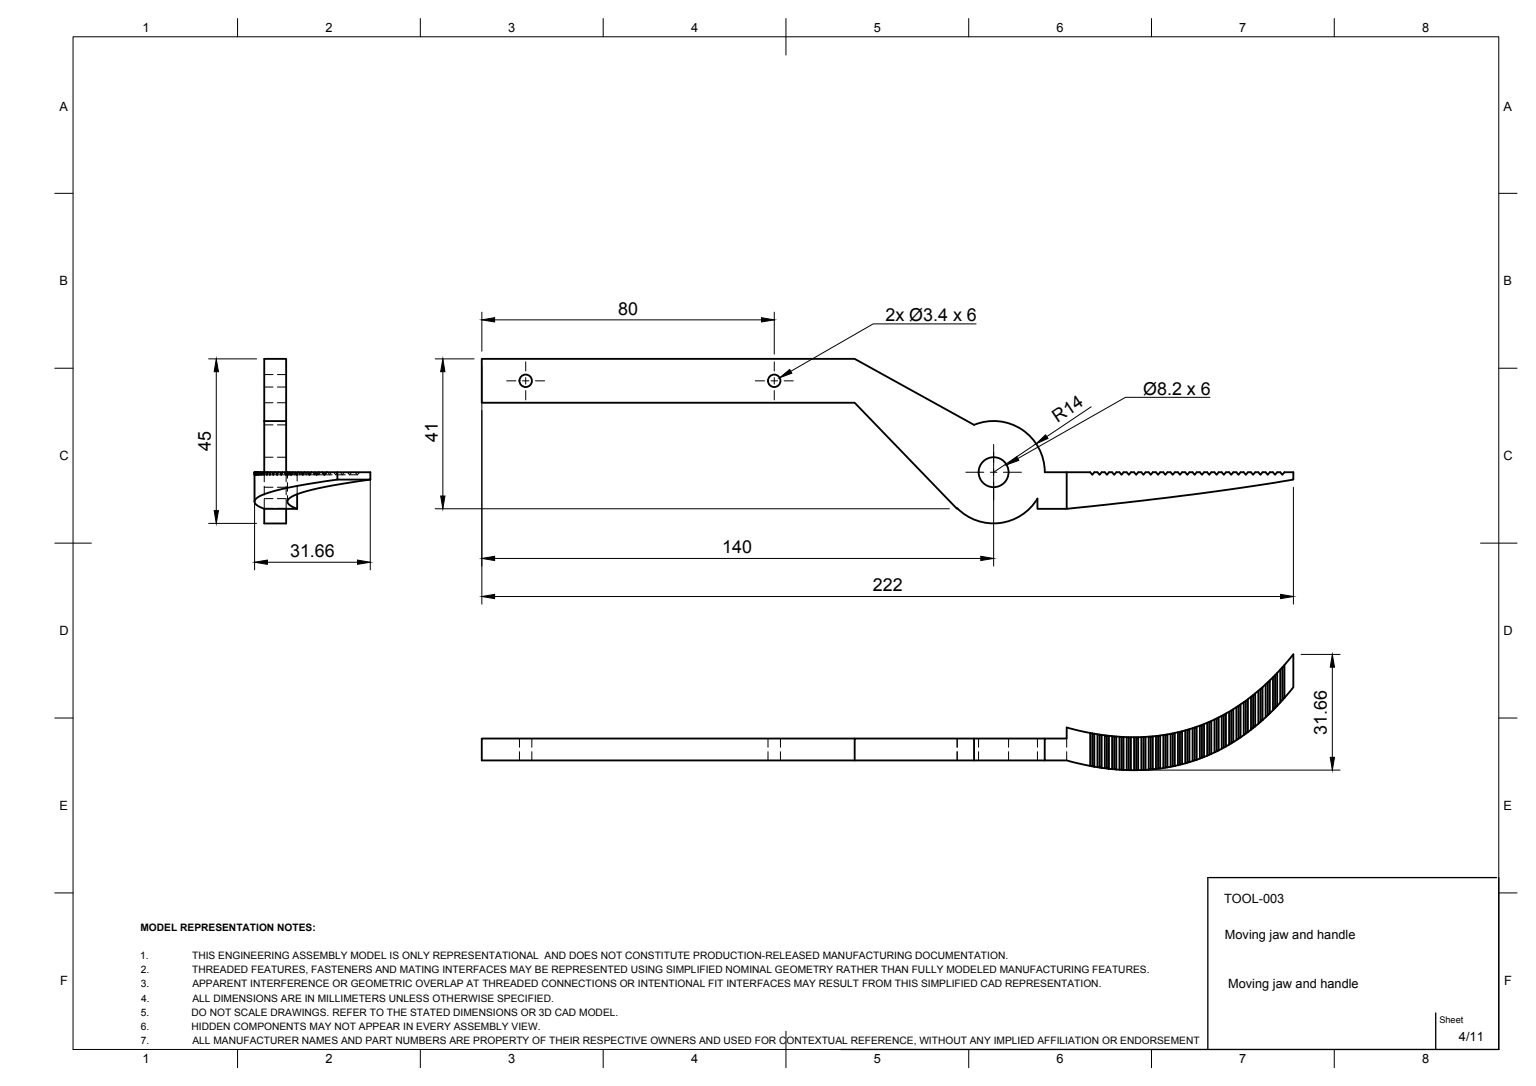
ISO-10303-21;
HEADER;
/* Generated by software containing ST-Developer
 * from STEP Tools, Inc. (www.steptools.com) 
 */

FILE_DESCRIPTION(
/* description */ (''),
/* implementation_level */ '2;1');

FILE_NAME(
/* name */ 'Moving jaw and handle.step',
/* time_stamp */ '2026-11-10T05:20:16-08:00',
/* author */ (''),
/* organization */ (''),
/* preprocessor_version */ 'ST-DEVELOPER v20.2',
/* originating_system */ 'Autodesk Translation Framework v15.17.0.0',
/* authorisation */ '');

FILE_SCHEMA (('AUTOMOTIVE_DESIGN { 1 0 10303 214 3 1 1 }'));
ENDSEC;

DATA;
#10=MECHANICAL_DESIGN_GEOMETRIC_PRESENTATION_REPRESENTATION('',(#113),#24809);
#93=SHAPE_REPRESENTATION_RELATIONSHIP('SRR','None',#24856,#103);
#103=ADVANCED_BREP_SHAPE_REPRESENTATION('',(#123),#24799);
#113=STYLED_ITEM('',(#24919),#123);
#123=MANIFOLD_SOLID_BREP('Body1',#9890);
#138=FACE_BOUND('',#2066,.T.);
#139=FACE_BOUND('',#2067,.T.);
#140=FACE_BOUND('',#2068,.T.);
#141=FACE_BOUND('',#2076,.T.);
#142=FACE_BOUND('',#2077,.T.);
#143=FACE_BOUND('',#2078,.T.);
#202=B_SPLINE_SURFACE_WITH_KNOTS('',3,3,((#14482,#14483,#14484,#14485),
(#14486,#14487,#14488,#14489),(#14490,#14491,#14492,#14493),(#14494,#14495,
#14496,#14497)),.UNSPECIFIED.,.F.,.F.,.F.,(4,4),(4,4),(0.,1.),(0.,1.),
 .UNSPECIFIED.);
#203=B_SPLINE_SURFACE_WITH_KNOTS('',3,3,((#14775,#14776,#14777,#14778),
(#14779,#14780,#14781,#14782),(#14783,#14784,#14785,#14786),(#14787,#14788,
#14789,#14790)),.UNSPECIFIED.,.F.,.F.,.F.,(4,4),(4,4),(0.,1.),(0.,1.),
 .UNSPECIFIED.);
#204=B_SPLINE_SURFACE_WITH_KNOTS('',3,3,((#14799,#14800,#14801,#14802),
(#14803,#14804,#14805,#14806),(#14807,#14808,#14809,#14810),(#14811,#14812,
#14813,#14814)),.UNSPECIFIED.,.F.,.F.,.F.,(4,4),(4,4),(0.,1.),(0.,1.),
 .UNSPECIFIED.);
#451=B_SPLINE_CURVE_WITH_KNOTS('',3,(#13756,#13757,#13758,#13759),
 .UNSPECIFIED.,.F.,.F.,(4,4),(-0.0905761996649145,0.),.UNSPECIFIED.);
#452=B_SPLINE_CURVE_WITH_KNOTS('',3,(#13763,#13764,#13765,#13766),
 .UNSPECIFIED.,.F.,.F.,(4,4),(-0.140808190495876,-0.0502319921300094),
 .UNSPECIFIED.);
#453=B_SPLINE_CURVE_WITH_KNOTS('',3,(#13770,#13771,#13772,#13773),
 .UNSPECIFIED.,.F.,.F.,(4,4),(-0.140839715426601,-0.050218000331002),
 .UNSPECIFIED.);
#454=B_SPLINE_CURVE_WITH_KNOTS('',3,(#13776,#13777,#13778,#13779),
 .UNSPECIFIED.,.F.,.F.,(4,4),(-0.0906217137909262,0.),.UNSPECIFIED.);
#455=B_SPLINE_CURVE_WITH_KNOTS('',3,(#13783,#13784,#13785,#13786),
 .UNSPECIFIED.,.F.,.F.,(4,4),(-0.0903212873282921,0.),.UNSPECIFIED.);
#456=B_SPLINE_CURVE_WITH_KNOTS('',3,(#13790,#13791,#13792,#13793),
 .UNSPECIFIED.,.F.,.F.,(4,4),(-0.140404708440305,-0.0500834223435583),
 .UNSPECIFIED.);
#457=B_SPLINE_CURVE_WITH_KNOTS('',3,(#13797,#13798,#13799,#13800),
 .UNSPECIFIED.,.F.,.F.,(4,4),(-0.14042464555609,-0.0500745698464118),
 .UNSPECIFIED.);
#458=B_SPLINE_CURVE_WITH_KNOTS('',3,(#13803,#13804,#13805,#13806),
 .UNSPECIFIED.,.F.,.F.,(4,4),(-0.0903500744707045,0.),.UNSPECIFIED.);
#459=B_SPLINE_CURVE_WITH_KNOTS('',3,(#13810,#13811,#13812,#13813),
 .UNSPECIFIED.,.F.,.F.,(4,4),(-0.0901993320901174,0.),.UNSPECIFIED.);
#460=B_SPLINE_CURVE_WITH_KNOTS('',3,(#13817,#13818,#13819,#13820),
 .UNSPECIFIED.,.F.,.F.,(4,4),(-0.140206191642939,-0.0500068606873887),
 .UNSPECIFIED.);
#461=B_SPLINE_CURVE_WITH_KNOTS('',3,(#13824,#13825,#13826,#13827),
 .UNSPECIFIED.,.F.,.F.,(4,4),(-0.14021182661721,-0.0500043514612263),
 .UNSPECIFIED.);
#462=B_SPLINE_CURVE_WITH_KNOTS('',3,(#13830,#13831,#13832,#13833),
 .UNSPECIFIED.,.F.,.F.,(4,4),(-0.0902074740142199,0.),.UNSPECIFIED.);
#463=B_SPLINE_CURVE_WITH_KNOTS('',3,(#13837,#13838,#13839,#13840),
 .UNSPECIFIED.,.F.,.F.,(4,4),(-0.0902411601010579,0.),.UNSPECIFIED.);
#464=B_SPLINE_CURVE_WITH_KNOTS('',3,(#13844,#13845,#13846,#13847),
 .UNSPECIFIED.,.F.,.F.,(4,4),(-0.140260192719421,-0.0500190336234041),
 .UNSPECIFIED.);
#465=B_SPLINE_CURVE_WITH_KNOTS('',3,(#13851,#13852,#13853,#13854),
 .UNSPECIFIED.,.F.,.F.,(4,4),(-0.140248231571563,-0.0500243288351115),
 .UNSPECIFIED.);
#466=B_SPLINE_CURVE_WITH_KNOTS('',3,(#13857,#13858,#13859,#13860),
 .UNSPECIFIED.,.F.,.F.,(4,4),(-0.0902239017224492,0.),.UNSPECIFIED.);
#467=B_SPLINE_CURVE_WITH_KNOTS('',3,(#13864,#13865,#13866,#13867),
 .UNSPECIFIED.,.F.,.F.,(4,4),(-0.090484186224837,0.),.UNSPECIFIED.);
#468=B_SPLINE_CURVE_WITH_KNOTS('',3,(#13871,#13872,#13873,#13874),
 .UNSPECIFIED.,.F.,.F.,(4,4),(-0.140624427659317,-0.0501402422817707),
 .UNSPECIFIED.);
#469=B_SPLINE_CURVE_WITH_KNOTS('',3,(#13878,#13879,#13880,#13881),
 .UNSPECIFIED.,.F.,.F.,(4,4),(-0.140590871945081,-0.0501551157110306),
 .UNSPECIFIED.);
#470=B_SPLINE_CURVE_WITH_KNOTS('',3,(#13884,#13885,#13886,#13887),
 .UNSPECIFIED.,.F.,.F.,(4,4),(-0.0904357553781669,0.),.UNSPECIFIED.);
#471=B_SPLINE_CURVE_WITH_KNOTS('',3,(#13891,#13892,#13893,#13894),
 .UNSPECIFIED.,.F.,.F.,(4,4),(-0.090973834374982,0.),.UNSPECIFIED.);
#472=B_SPLINE_CURVE_WITH_KNOTS('',3,(#13898,#13899,#13900,#13901),
 .UNSPECIFIED.,.F.,.F.,(4,4),(-0.141368966615449,-0.0503951329062475),
 .UNSPECIFIED.);
#473=B_SPLINE_CURVE_WITH_KNOTS('',3,(#13905,#13906,#13907,#13908),
 .UNSPECIFIED.,.F.,.F.,(4,4),(-0.141308961367084,-0.0504217384669459),
 .UNSPECIFIED.);
#474=B_SPLINE_CURVE_WITH_KNOTS('',3,(#13911,#13912,#13913,#13914),
 .UNSPECIFIED.,.F.,.F.,(4,4),(-0.0908872222229066,0.),.UNSPECIFIED.);
#475=B_SPLINE_CURVE_WITH_KNOTS('',3,(#13918,#13919,#13920,#13921),
 .UNSPECIFIED.,.F.,.F.,(4,4),(-0.110639644983061,0.),.UNSPECIFIED.);
#476=B_SPLINE_CURVE_WITH_KNOTS('',3,(#13925,#13926,#13927,#13928),
 .UNSPECIFIED.,.F.,.F.,(4,4),(-0.171616644636876,-0.0609769995431898),
 .UNSPECIFIED.);
#477=B_SPLINE_CURVE_WITH_KNOTS('',3,(#13932,#13933,#13934,#13935),
 .UNSPECIFIED.,.F.,.F.,(4,4),(-0.171044536664633,-0.0612308128915547),
 .UNSPECIFIED.);
#478=B_SPLINE_CURVE_WITH_KNOTS('',3,(#13938,#13939,#13940,#13941),
 .UNSPECIFIED.,.F.,.F.,(4,4),(-0.109813723871753,0.),.UNSPECIFIED.);
#479=B_SPLINE_CURVE_WITH_KNOTS('',3,(#13945,#13946,#13947,#13948),
 .UNSPECIFIED.,.F.,.F.,(4,4),(-0.0922945850422147,0.),.UNSPECIFIED.);
#480=B_SPLINE_CURVE_WITH_KNOTS('',3,(#13952,#13953,#13954,#13955),
 .UNSPECIFIED.,.F.,.F.,(4,4),(-0.143389908932554,-0.0510953242730707),
 .UNSPECIFIED.);
#481=B_SPLINE_CURVE_WITH_KNOTS('',3,(#13959,#13960,#13961,#13962),
 .UNSPECIFIED.,.F.,.F.,(4,4),(-0.143278783493244,-0.0511446064988726),
 .UNSPECIFIED.);
#482=B_SPLINE_CURVE_WITH_KNOTS('',3,(#13965,#13966,#13967,#13968),
 .UNSPECIFIED.,.F.,.F.,(4,4),(-0.0921341766004976,0.),.UNSPECIFIED.);
#483=B_SPLINE_CURVE_WITH_KNOTS('',3,(#13972,#13973,#13974,#13975),
 .UNSPECIFIED.,.F.,.F.,(4,4),(-0.0936688606535915,0.),.UNSPECIFIED.);
#484=B_SPLINE_CURVE_WITH_KNOTS('',3,(#13979,#13980,#13981,#13982),
 .UNSPECIFIED.,.F.,.F.,(4,4),(-0.145498716334213,-0.0518298558949936),
 .UNSPECIFIED.);
#485=B_SPLINE_CURVE_WITH_KNOTS('',3,(#13986,#13987,#13988,#13989),
 .UNSPECIFIED.,.F.,.F.,(4,4),(-0.145343920697893,-0.0518985113244783),
 .UNSPECIFIED.);
#486=B_SPLINE_CURVE_WITH_KNOTS('',3,(#13992,#13993,#13994,#13995),
 .UNSPECIFIED.,.F.,.F.,(4,4),(-0.0934454091497814,0.),.UNSPECIFIED.);
#487=B_SPLINE_CURVE_WITH_KNOTS('',3,(#13999,#14000,#14001,#14002),
 .UNSPECIFIED.,.F.,.F.,(4,4),(-0.0955408943961818,0.),.UNSPECIFIED.);
#488=B_SPLINE_CURVE_WITH_KNOTS('',3,(#14006,#14007,#14008,#14009),
 .UNSPECIFIED.,.F.,.F.,(4,4),(-0.148375189783694,-0.0528342954751738),
 .UNSPECIFIED.);
#489=B_SPLINE_CURVE_WITH_KNOTS('',3,(#14013,#14014,#14015,#14016),
 .UNSPECIFIED.,.F.,.F.,(4,4),(-0.148167070467038,-0.0529266079685813),
 .UNSPECIFIED.);
#490=B_SPLINE_CURVE_WITH_KNOTS('',3,(#14019,#14020,#14021,#14022),
 .UNSPECIFIED.,.F.,.F.,(4,4),(-0.0952404624045437,0.),.UNSPECIFIED.);
#491=B_SPLINE_CURVE_WITH_KNOTS('',3,(#14026,#14027,#14028,#14029),
 .UNSPECIFIED.,.F.,.F.,(4,4),(-0.0980208974210048,0.),.UNSPECIFIED.);
#492=B_SPLINE_CURVE_WITH_KNOTS('',3,(#14033,#14034,#14035,#14036),
 .UNSPECIFIED.,.F.,.F.,(4,4),(-0.152189280292737,-0.0541683828893004),
 .UNSPECIFIED.);
#493=B_SPLINE_CURVE_WITH_KNOTS('',3,(#14040,#14041,#14042,#14043),
 .UNSPECIFIED.,.F.,.F.,(4,4),(-0.151916008013229,-0.0542896020155086),
 .UNSPECIFIED.);
#494=B_SPLINE_CURVE_WITH_KNOTS('',3,(#14046,#14047,#14048,#14049),
 .UNSPECIFIED.,.F.,.F.,(4,4),(-0.0976264059776055,0.),.UNSPECIFIED.);
#495=B_SPLINE_CURVE_WITH_KNOTS('',3,(#14053,#14054,#14055,#14056),
 .UNSPECIFIED.,.F.,.F.,(4,4),(-0.101244462273373,0.),.UNSPECIFIED.);
#496=B_SPLINE_CURVE_WITH_KNOTS('',3,(#14060,#14061,#14062,#14063),
 .UNSPECIFIED.,.F.,.F.,(4,4),(-0.157150018704206,-0.0559055564306627),
 .UNSPECIFIED.);
#497=B_SPLINE_CURVE_WITH_KNOTS('',3,(#14067,#14068,#14069,#14070),
 .UNSPECIFIED.,.F.,.F.,(4,4),(-0.156796992217562,-0.056062161879322),
 .UNSPECIFIED.);
#498=B_SPLINE_CURVE_WITH_KNOTS('',3,(#14073,#14074,#14075,#14076),
 .UNSPECIFIED.,.F.,.F.,(4,4),(-0.100734830337421,0.),.UNSPECIFIED.);
#499=B_SPLINE_CURVE_WITH_KNOTS('',3,(#14080,#14081,#14082,#14083),
 .UNSPECIFIED.,.F.,.F.,(4,4),(-0.10537999886802,0.),.UNSPECIFIED.);
#500=B_SPLINE_CURVE_WITH_KNOTS('',3,(#14087,#14088,#14089,#14090),
 .UNSPECIFIED.,.F.,.F.,(4,4),(-0.163516913195776,-0.058136914319678),
 .UNSPECIFIED.);
#501=B_SPLINE_CURVE_WITH_KNOTS('',3,(#14094,#14095,#14096,#14097),
 .UNSPECIFIED.,.F.,.F.,(4,4),(-0.163065906917568,-0.0583369938462544),
 .UNSPECIFIED.);
#502=B_SPLINE_CURVE_WITH_KNOTS('',3,(#14100,#14101,#14102,#14103),
 .UNSPECIFIED.,.F.,.F.,(4,4),(-0.104728913077325,0.),.UNSPECIFIED.);
#503=B_SPLINE_CURVE_WITH_KNOTS('',3,(#14107,#14108,#14109,#14110),
 .UNSPECIFIED.,.F.,.F.,(4,4),(-0.1078539391682,0.),.UNSPECIFIED.);
#504=B_SPLINE_CURVE_WITH_KNOTS('',3,(#14114,#14115,#14116,#14117),
 .UNSPECIFIED.,.F.,.F.,(4,4),(-0.167326517821918,-0.0594725786155369),
 .UNSPECIFIED.);
#505=B_SPLINE_CURVE_WITH_KNOTS('',3,(#14121,#14122,#14123,#14124),
 .UNSPECIFIED.,.F.,.F.,(4,4),(-0.16681822317347,-0.0596980774786193),
 .UNSPECIFIED.);
#506=B_SPLINE_CURVE_WITH_KNOTS('',3,(#14127,#14128,#14129,#14130),
 .UNSPECIFIED.,.F.,.F.,(4,4),(-0.107120145727053,0.),.UNSPECIFIED.);
#507=B_SPLINE_CURVE_WITH_KNOTS('',3,(#14134,#14135,#14136,#14137),
 .UNSPECIFIED.,.F.,.F.,(4,4),(-0.103186160248021,0.),.UNSPECIFIED.);
#508=B_SPLINE_CURVE_WITH_KNOTS('',3,(#14141,#14142,#14143,#14144),
 .UNSPECIFIED.,.F.,.F.,(4,4),(-0.160139097703419,-0.0569529374542383),
 .UNSPECIFIED.);
#509=B_SPLINE_CURVE_WITH_KNOTS('',3,(#14148,#14149,#14150,#14151),
 .UNSPECIFIED.,.F.,.F.,(4,4),(-0.159739629262513,-0.0571301493054397),
 .UNSPECIFIED.);
#510=B_SPLINE_CURVE_WITH_KNOTS('',3,(#14154,#14155,#14156,#14157),
 .UNSPECIFIED.,.F.,.F.,(4,4),(-0.102609479957307,0.),.UNSPECIFIED.);
#511=B_SPLINE_CURVE_WITH_KNOTS('',3,(#14161,#14162,#14163,#14164),
 .UNSPECIFIED.,.F.,.F.,(4,4),(-0.0995300847676173,0.),.UNSPECIFIED.);
#512=B_SPLINE_CURVE_WITH_KNOTS('',3,(#14168,#14169,#14170,#14171),
 .UNSPECIFIED.,.F.,.F.,(4,4),(-0.154511445578318,-0.0549813608126789),
 .UNSPECIFIED.);
#513=B_SPLINE_CURVE_WITH_KNOTS('',3,(#14175,#14176,#14177,#14178),
 .UNSPECIFIED.,.F.,.F.,(4,4),(-0.154200323996305,-0.0551193732220978),
 .UNSPECIFIED.);
#514=B_SPLINE_CURVE_WITH_KNOTS('',3,(#14181,#14182,#14183,#14184),
 .UNSPECIFIED.,.F.,.F.,(4,4),(-0.0990809507692,0.),.UNSPECIFIED.);
#515=B_SPLINE_CURVE_WITH_KNOTS('',3,(#14188,#14189,#14190,#14191),
 .UNSPECIFIED.,.F.,.F.,(4,4),(-0.096697094267499,0.),.UNSPECIFIED.);
#516=B_SPLINE_CURVE_WITH_KNOTS('',3,(#14195,#14196,#14197,#14198),
 .UNSPECIFIED.,.F.,.F.,(4,4),(-0.150152998198254,-0.0534559039759521),
 .UNSPECIFIED.);
#517=B_SPLINE_CURVE_WITH_KNOTS('',3,(#14202,#14203,#14204,#14205),
 .UNSPECIFIED.,.F.,.F.,(4,4),(-0.14991393792459,-0.0535619439725345),
 .UNSPECIFIED.);
#518=B_SPLINE_CURVE_WITH_KNOTS('',3,(#14208,#14209,#14210,#14211),
 .UNSPECIFIED.,.F.,.F.,(4,4),(-0.0963519939024695,0.),.UNSPECIFIED.);
#519=B_SPLINE_CURVE_WITH_KNOTS('',3,(#14215,#14216,#14217,#14218),
 .UNSPECIFIED.,.F.,.F.,(4,4),(-0.0945362942895881,0.),.UNSPECIFIED.);
#520=B_SPLINE_CURVE_WITH_KNOTS('',3,(#14222,#14223,#14224,#14225),
 .UNSPECIFIED.,.F.,.F.,(4,4),(-0.14683118116155,-0.0522948870165077),
 .UNSPECIFIED.);
#521=B_SPLINE_CURVE_WITH_KNOTS('',3,(#14229,#14230,#14231,#14232),
 .UNSPECIFIED.,.F.,.F.,(4,4),(-0.146651054618532,-0.0523747803462794),
 .UNSPECIFIED.);
#522=B_SPLINE_CURVE_WITH_KNOTS('',3,(#14235,#14236,#14237,#14238),
 .UNSPECIFIED.,.F.,.F.,(4,4),(-0.094276274119846,0.),.UNSPECIFIED.);
#523=B_SPLINE_CURVE_WITH_KNOTS('',3,(#14242,#14243,#14244,#14245),
 .UNSPECIFIED.,.F.,.F.,(4,4),(-0.092925555225633,0.),.UNSPECIFIED.);
#524=B_SPLINE_CURVE_WITH_KNOTS('',3,(#14249,#14250,#14251,#14252),
 .UNSPECIFIED.,.F.,.F.,(4,4),(-0.144357688280225,-0.0514321333491983),
 .UNSPECIFIED.);
#525=B_SPLINE_CURVE_WITH_KNOTS('',3,(#14256,#14257,#14258,#14259),
 .UNSPECIFIED.,.F.,.F.,(4,4),(-0.144225816874814,-0.0514906188728281),
 .UNSPECIFIED.);
#526=B_SPLINE_CURVE_WITH_KNOTS('',3,(#14262,#14263,#14264,#14265),
 .UNSPECIFIED.,.F.,.F.,(4,4),(-0.0927351976969034,0.),.UNSPECIFIED.);
#527=B_SPLINE_CURVE_WITH_KNOTS('',3,(#14269,#14270,#14271,#14272),
 .UNSPECIFIED.,.F.,.F.,(4,4),(-0.0917652731638768,0.),.UNSPECIFIED.);
#528=B_SPLINE_CURVE_WITH_KNOTS('',3,(#14276,#14277,#14278,#14279),
 .UNSPECIFIED.,.F.,.F.,(4,4),(-0.142578910435786,-0.0508136377474404),
 .UNSPECIFIED.);
#529=B_SPLINE_CURVE_WITH_KNOTS('',3,(#14283,#14284,#14285,#14286),
 .UNSPECIFIED.,.F.,.F.,(4,4),(-0.142486557842336,-0.0508545922219399),
 .UNSPECIFIED.);
#530=B_SPLINE_CURVE_WITH_KNOTS('',3,(#14289,#14290,#14291,#14292),
 .UNSPECIFIED.,.F.,.F.,(4,4),(-0.0916319651330652,0.),.UNSPECIFIED.);
#531=B_SPLINE_CURVE_WITH_KNOTS('',3,(#14296,#14297,#14298,#14299),
 .UNSPECIFIED.,.F.,.F.,(4,4),(-0.0913279460148378,0.),.UNSPECIFIED.);
#532=B_SPLINE_CURVE_WITH_KNOTS('',3,(#14303,#14304,#14305,#14306),
 .UNSPECIFIED.,.F.,.F.,(4,4),(-0.141909771824219,-0.0505818263802296),
 .UNSPECIFIED.);
#533=B_SPLINE_CURVE_WITH_KNOTS('',3,(#14310,#14311,#14312,#14313),
 .UNSPECIFIED.,.F.,.F.,(4,4),(-0.141834403711857,-0.0506152466388435),
 .UNSPECIFIED.);
#534=B_SPLINE_CURVE_WITH_KNOTS('',3,(#14316,#14317,#14318,#14319),
 .UNSPECIFIED.,.F.,.F.,(4,4),(-0.0912191564904243,0.),.UNSPECIFIED.);
#535=B_SPLINE_CURVE_WITH_KNOTS('',3,(#14323,#14324,#14325,#14326),
 .UNSPECIFIED.,.F.,.F.,(4,4),(-0.0906949857339717,0.),.UNSPECIFIED.);
#536=B_SPLINE_CURVE_WITH_KNOTS('',3,(#14330,#14331,#14332,#14333),
 .UNSPECIFIED.,.F.,.F.,(4,4),(-0.140944227820591,-0.0502492428443703),
 .UNSPECIFIED.);
#537=B_SPLINE_CURVE_WITH_KNOTS('',3,(#14337,#14338,#14339,#14340),
 .UNSPECIFIED.,.F.,.F.,(4,4),(-0.140898114560254,-0.0502696863145455),
 .UNSPECIFIED.);
#538=B_SPLINE_CURVE_WITH_KNOTS('',3,(#14343,#14344,#14345,#14346),
 .UNSPECIFIED.,.F.,.F.,(4,4),(-0.0906284274757685,0.),.UNSPECIFIED.);
#539=B_SPLINE_CURVE_WITH_KNOTS('',3,(#14350,#14351,#14352,#14353),
 .UNSPECIFIED.,.F.,.F.,(4,4),(-0.0903348907359758,0.),.UNSPECIFIED.);
#540=B_SPLINE_CURVE_WITH_KNOTS('',3,(#14357,#14358,#14359,#14360),
 .UNSPECIFIED.,.F.,.F.,(4,4),(-0.140399469840189,-0.0500645800333094),
 .UNSPECIFIED.);
#541=B_SPLINE_CURVE_WITH_KNOTS('',3,(#14364,#14365,#14366,#14367),
 .UNSPECIFIED.,.F.,.F.,(4,4),(-0.140377260822424,-0.0500744206159611),
 .UNSPECIFIED.);
#542=B_SPLINE_CURVE_WITH_KNOTS('',3,(#14370,#14371,#14372,#14373),
 .UNSPECIFIED.,.F.,.F.,(4,4),(-0.0903028392675632,0.),.UNSPECIFIED.);
#543=B_SPLINE_CURVE_WITH_KNOTS('',3,(#14377,#14378,#14379,#14380),
 .UNSPECIFIED.,.F.,.F.,(4,4),(-0.0901976044608984,0.),.UNSPECIFIED.);
#544=B_SPLINE_CURVE_WITH_KNOTS('',3,(#14384,#14385,#14386,#14387),
 .UNSPECIFIED.,.F.,.F.,(4,4),(-0.140198281967887,-0.050000678580588),
 .UNSPECIFIED.);
#545=B_SPLINE_CURVE_WITH_KNOTS('',3,(#14391,#14392,#14393,#14394),
 .UNSPECIFIED.,.F.,.F.,(4,4),(-0.14019557144157,-0.0500018708171553),
 .UNSPECIFIED.);
#546=B_SPLINE_CURVE_WITH_KNOTS('',3,(#14397,#14398,#14399,#14400),
 .UNSPECIFIED.,.F.,.F.,(4,4),(-0.0901936995426637,0.),.UNSPECIFIED.);
#547=B_SPLINE_CURVE_WITH_KNOTS('',3,(#14404,#14405,#14406,#14407),
 .UNSPECIFIED.,.F.,.F.,(4,4),(-0.090241903072294,0.),.UNSPECIFIED.);
#548=B_SPLINE_CURVE_WITH_KNOTS('',3,(#14411,#14412,#14413,#14414),
 .UNSPECIFIED.,.F.,.F.,(4,4),(-0.140277072739373,-0.0500351708536283),
 .UNSPECIFIED.);
#549=B_SPLINE_CURVE_WITH_KNOTS('',3,(#14418,#14419,#14420,#14421),
 .UNSPECIFIED.,.F.,.F.,(4,4),(-0.14029023165943,-0.0500293245949378),
 .UNSPECIFIED.);
#550=B_SPLINE_CURVE_WITH_KNOTS('',3,(#14424,#14425,#14426,#14427),
 .UNSPECIFIED.,.F.,.F.,(4,4),(-0.0902609058696926,0.),.UNSPECIFIED.);
#551=B_SPLINE_CURVE_WITH_KNOTS('',3,(#14431,#14432,#14433,#14434),
 .UNSPECIFIED.,.F.,.F.,(4,4),(-0.0904338265476047,0.),.UNSPECIFIED.);
#552=B_SPLINE_CURVE_WITH_KNOTS('',3,(#14438,#14439,#14440,#14441),
 .UNSPECIFIED.,.F.,.F.,(4,4),(-0.140583455402597,-0.050149630123983),
 .UNSPECIFIED.);
#553=B_SPLINE_CURVE_WITH_KNOTS('',3,(#14445,#14446,#14447,#14448),
 .UNSPECIFIED.,.F.,.F.,(4,4),(-0.140609493729256,-0.0501380716718544),
 .UNSPECIFIED.);
#554=B_SPLINE_CURVE_WITH_KNOTS('',3,(#14451,#14452,#14453,#14454),
 .UNSPECIFIED.,.F.,.F.,(4,4),(-0.0904714207818447,0.),.UNSPECIFIED.);
#555=B_SPLINE_CURVE_WITH_KNOTS('',3,(#14458,#14459,#14460,#14461),
 .UNSPECIFIED.,.F.,.F.,(4,4),(-0.0907453915343808,0.),.UNSPECIFIED.);
#556=B_SPLINE_CURVE_WITH_KNOTS('',3,(#14465,#14466,#14467,#14468),
 .UNSPECIFIED.,.F.,.F.,(4,4),(-0.141074262480741,-0.0503288722684034),
 .UNSPECIFIED.);
#557=B_SPLINE_CURVE_WITH_KNOTS('',3,(#14472,#14473,#14474,#14475),
 .UNSPECIFIED.,.F.,.F.,(4,4),(-0.141110715992304,-0.0503126946273584),
 .UNSPECIFIED.);
#558=B_SPLINE_CURVE_WITH_KNOTS('',3,(#14478,#14479,#14480,#14481),
 .UNSPECIFIED.,.F.,.F.,(4,4),(-0.0907980200379908,0.),.UNSPECIFIED.);
#559=B_SPLINE_CURVE_WITH_KNOTS('',3,(#14498,#14499,#14500,#14501),
 .UNSPECIFIED.,.F.,.F.,(4,4),(0.129763535305857,0.141771498582774),
 .UNSPECIFIED.);
#560=B_SPLINE_CURVE_WITH_KNOTS('',3,(#14502,#14503,#14504,#14505),
 .UNSPECIFIED.,.F.,.F.,(4,4),(0.157691595007123,0.169827160768426),
 .UNSPECIFIED.);
#561=B_SPLINE_CURVE_WITH_KNOTS('',3,(#14506,#14507,#14508,#14509),
 .UNSPECIFIED.,.F.,.F.,(4,4),(0.185918250377541,0.198185574966566),
 .UNSPECIFIED.);
#562=B_SPLINE_CURVE_WITH_KNOTS('',3,(#14510,#14511,#14512,#14513),
 .UNSPECIFIED.,.F.,.F.,(4,4),(0.214453288668711,0.226856759081898),
 .UNSPECIFIED.);
#563=B_SPLINE_CURVE_WITH_KNOTS('',3,(#14514,#14515,#14516,#14517),
 .UNSPECIFIED.,.F.,.F.,(4,4),(0.243307043781977,0.255851295996116),
 .UNSPECIFIED.);
#564=B_SPLINE_CURVE_WITH_KNOTS('',3,(#14518,#14519,#14520,#14521),
 .UNSPECIFIED.,.F.,.F.,(4,4),(0.272490439993122,0.28518037920845),
 .UNSPECIFIED.);
#565=B_SPLINE_CURVE_WITH_KNOTS('',3,(#14522,#14523,#14524,#14525),
 .UNSPECIFIED.,.F.,.F.,(4,4),(0.302015040279167,0.314855863328957),
 .UNSPECIFIED.);
#566=B_SPLINE_CURVE_WITH_KNOTS('',3,(#14526,#14527,#14528,#14529),
 .UNSPECIFIED.,.F.,.F.,(4,4),(0.33189309985356,0.344890320070497),
 .UNSPECIFIED.);
#567=B_SPLINE_CURVE_WITH_KNOTS('',3,(#14530,#14531,#14532,#14533),
 .UNSPECIFIED.,.F.,.F.,(4,4),(0.362137625612687,0.375297100489449),
 .UNSPECIFIED.);
#568=B_SPLINE_CURVE_WITH_KNOTS('',3,(#14534,#14535,#14536,#14537),
 .UNSPECIFIED.,.F.,.F.,(4,4),(0.392762442311623,0.406090404349278),
 .UNSPECIFIED.);
#569=B_SPLINE_CURVE_WITH_KNOTS('',3,(#14538,#14539,#14540,#14541),
 .UNSPECIFIED.,.F.,.F.,(4,4),(0.423782266424232,0.437285357629296),
 .UNSPECIFIED.);
#570=B_SPLINE_CURVE_WITH_KNOTS('',3,(#14542,#14543,#14544,#14545),
 .UNSPECIFIED.,.F.,.F.,(4,4),(0.455212788807218,0.468898099379087),
 .UNSPECIFIED.);
#571=B_SPLINE_CURVE_WITH_KNOTS('',3,(#14546,#14547,#14548,#14549),
 .UNSPECIFIED.,.F.,.F.,(4,4),(0.48707076748574,0.500945879333897),
 .UNSPECIFIED.);
#572=B_SPLINE_CURVE_WITH_KNOTS('',3,(#14550,#14551,#14552,#14553),
 .UNSPECIFIED.,.F.,.F.,(4,4),(0.519374132117822,0.533447167966844),
 .UNSPECIFIED.);
#573=B_SPLINE_CURVE_WITH_KNOTS('',3,(#14554,#14555,#14556,#14557),
 .UNSPECIFIED.,.F.,.F.,(4,4),(0.55214210198613,0.566421780971217),
 .UNSPECIFIED.);
#574=B_SPLINE_CURVE_WITH_KNOTS('',3,(#14558,#14559,#14560,#14561),
 .UNSPECIFIED.,.F.,.F.,(4,4),(0.585395319721713,0.599891020555078),
 .UNSPECIFIED.);
#575=B_SPLINE_CURVE_WITH_KNOTS('',3,(#14562,#14563,#14564,#14565),
 .UNSPECIFIED.,.F.,.F.,(4,4),(0.619156003402013,0.633877836409608),
 .UNSPECIFIED.);
#576=B_SPLINE_CURVE_WITH_KNOTS('',3,(#14566,#14567,#14568,#14569),
 .UNSPECIFIED.,.F.,.F.,(4,4),(0.653448120206462,0.668407009806632),
 .UNSPECIFIED.);
#577=B_SPLINE_CURVE_WITH_KNOTS('',3,(#14570,#14571,#14572,#14573),
 .UNSPECIFIED.,.F.,.F.,(4,4),(0.688297585486082,0.703505365021776),
 .UNSPECIFIED.);
#578=B_SPLINE_CURVE_WITH_KNOTS('',3,(#14574,#14575,#14576,#14577),
 .UNSPECIFIED.,.F.,.F.,(4,4),(0.723732491946339,0.739202013210385),
 .UNSPECIFIED.);
#579=B_SPLINE_CURVE_WITH_KNOTS('',3,(#14578,#14579,#14580,#14581),
 .UNSPECIFIED.,.F.,.F.,(4,4),(0.759783374705264,0.775528635040521),
 .UNSPECIFIED.);
#580=B_SPLINE_CURVE_WITH_KNOTS('',3,(#14582,#14583,#14584,#14585),
 .UNSPECIFIED.,.F.,.F.,(4,4),(0.796483519339086,0.812519809888056),
 .UNSPECIFIED.);
#581=B_SPLINE_CURVE_WITH_KNOTS('',3,(#14586,#14587,#14588,#14589),
 .UNSPECIFIED.,.F.,.F.,(4,4),(0.833869321756548,0.850213401327293),
 .UNSPECIFIED.);
#582=B_SPLINE_CURVE_WITH_KNOTS('',3,(#14590,#14591,#14592,#14593),
 .UNSPECIFIED.,.F.,.F.,(4,4),(0.87198071097596,0.888651011150777),
 .UNSPECIFIED.);
#583=B_SPLINE_CURVE_WITH_KNOTS('',3,(#14594,#14595,#14596,#14597),
 .UNSPECIFIED.,.F.,.F.,(4,4),(0.910861648789003,0.927878517423714),
 .UNSPECIFIED.);
#584=B_SPLINE_CURVE_WITH_KNOTS('',3,(#14599,#14600,#14601,#14602),
 .UNSPECIFIED.,.F.,.F.,(4,4),(0.950560724124997,1.),.UNSPECIFIED.);
#585=B_SPLINE_CURVE_WITH_KNOTS('',3,(#14606,#14607,#14608,#14609,#14610,
#14611),.UNSPECIFIED.,.F.,.F.,(4,2,4),(0.,0.510141450492869,1.),
 .UNSPECIFIED.);
#586=B_SPLINE_CURVE_WITH_KNOTS('',3,(#14614,#14615,#14616,#14617),
 .UNSPECIFIED.,.F.,.F.,(4,4),(0.,0.0865309392501863),.UNSPECIFIED.);
#587=B_SPLINE_CURVE_WITH_KNOTS('',3,(#14618,#14619,#14620,#14621),
 .UNSPECIFIED.,.F.,.F.,(4,4),(0.102124791024766,0.114009094135949),
 .UNSPECIFIED.);
#588=B_SPLINE_CURVE_WITH_KNOTS('',3,(#14624,#14625,#14626,#14627),
 .UNSPECIFIED.,.F.,.F.,(4,4),(0.950560724124998,1.),.UNSPECIFIED.);
#589=B_SPLINE_CURVE_WITH_KNOTS('',3,(#14638,#14639,#14640,#14641),
 .UNSPECIFIED.,.F.,.F.,(4,4),(0.,0.0865309392501863),.UNSPECIFIED.);
#590=B_SPLINE_CURVE_WITH_KNOTS('',3,(#14643,#14644,#14645,#14646),
 .UNSPECIFIED.,.F.,.F.,(4,4),(0.129763535305857,0.141771498582774),
 .UNSPECIFIED.);
#591=B_SPLINE_CURVE_WITH_KNOTS('',3,(#14648,#14649,#14650,#14651),
 .UNSPECIFIED.,.F.,.F.,(4,4),(0.185918250377541,0.198185574966566),
 .UNSPECIFIED.);
#592=B_SPLINE_CURVE_WITH_KNOTS('',3,(#14653,#14654,#14655,#14656),
 .UNSPECIFIED.,.F.,.F.,(4,4),(0.243307043781977,0.255851295996116),
 .UNSPECIFIED.);
#593=B_SPLINE_CURVE_WITH_KNOTS('',3,(#14658,#14659,#14660,#14661),
 .UNSPECIFIED.,.F.,.F.,(4,4),(0.302015040279167,0.314855863328958),
 .UNSPECIFIED.);
#594=B_SPLINE_CURVE_WITH_KNOTS('',3,(#14663,#14664,#14665,#14666),
 .UNSPECIFIED.,.F.,.F.,(4,4),(0.362137625612687,0.375297100489449),
 .UNSPECIFIED.);
#595=B_SPLINE_CURVE_WITH_KNOTS('',3,(#14668,#14669,#14670,#14671),
 .UNSPECIFIED.,.F.,.F.,(4,4),(0.423782266424232,0.437285357629297),
 .UNSPECIFIED.);
#596=B_SPLINE_CURVE_WITH_KNOTS('',3,(#14673,#14674,#14675,#14676),
 .UNSPECIFIED.,.F.,.F.,(4,4),(0.455212788807218,0.468898099379087),
 .UNSPECIFIED.);
#597=B_SPLINE_CURVE_WITH_KNOTS('',3,(#14678,#14679,#14680,#14681),
 .UNSPECIFIED.,.F.,.F.,(4,4),(0.519374132117822,0.533447167966844),
 .UNSPECIFIED.);
#598=B_SPLINE_CURVE_WITH_KNOTS('',3,(#14683,#14684,#14685,#14686),
 .UNSPECIFIED.,.F.,.F.,(4,4),(0.585395319721713,0.599891020555078),
 .UNSPECIFIED.);
#599=B_SPLINE_CURVE_WITH_KNOTS('',3,(#14688,#14689,#14690,#14691),
 .UNSPECIFIED.,.F.,.F.,(4,4),(0.653448120206462,0.668407009806632),
 .UNSPECIFIED.);
#600=B_SPLINE_CURVE_WITH_KNOTS('',3,(#14693,#14694,#14695,#14696),
 .UNSPECIFIED.,.F.,.F.,(4,4),(0.723732491946339,0.739202013210385),
 .UNSPECIFIED.);
#601=B_SPLINE_CURVE_WITH_KNOTS('',3,(#14698,#14699,#14700,#14701),
 .UNSPECIFIED.,.F.,.F.,(4,4),(0.796483519339086,0.812519809888056),
 .UNSPECIFIED.);
#602=B_SPLINE_CURVE_WITH_KNOTS('',3,(#14703,#14704,#14705,#14706),
 .UNSPECIFIED.,.F.,.F.,(4,4),(0.87198071097596,0.888651011150777),
 .UNSPECIFIED.);
#603=B_SPLINE_CURVE_WITH_KNOTS('',3,(#14708,#14709,#14710,#14711),
 .UNSPECIFIED.,.F.,.F.,(4,4),(0.833869321756548,0.850213401327293),
 .UNSPECIFIED.);
#604=B_SPLINE_CURVE_WITH_KNOTS('',3,(#14713,#14714,#14715,#14716),
 .UNSPECIFIED.,.F.,.F.,(4,4),(0.759783374705264,0.775528635040521),
 .UNSPECIFIED.);
#605=B_SPLINE_CURVE_WITH_KNOTS('',3,(#14718,#14719,#14720,#14721),
 .UNSPECIFIED.,.F.,.F.,(4,4),(0.688297585486082,0.703505365021776),
 .UNSPECIFIED.);
#606=B_SPLINE_CURVE_WITH_KNOTS('',3,(#14723,#14724,#14725,#14726),
 .UNSPECIFIED.,.F.,.F.,(4,4),(0.619156003402013,0.633877836409608),
 .UNSPECIFIED.);
#607=B_SPLINE_CURVE_WITH_KNOTS('',3,(#14728,#14729,#14730,#14731),
 .UNSPECIFIED.,.F.,.F.,(4,4),(0.55214210198613,0.566421780971217),
 .UNSPECIFIED.);
#608=B_SPLINE_CURVE_WITH_KNOTS('',3,(#14733,#14734,#14735,#14736),
 .UNSPECIFIED.,.F.,.F.,(4,4),(0.48707076748574,0.500945879333897),
 .UNSPECIFIED.);
#609=B_SPLINE_CURVE_WITH_KNOTS('',3,(#14738,#14739,#14740,#14741),
 .UNSPECIFIED.,.F.,.F.,(4,4),(0.910861648789003,0.927878517423714),
 .UNSPECIFIED.);
#610=B_SPLINE_CURVE_WITH_KNOTS('',3,(#14743,#14744,#14745,#14746),
 .UNSPECIFIED.,.F.,.F.,(4,4),(0.392762442311622,0.406090404349278),
 .UNSPECIFIED.);
#611=B_SPLINE_CURVE_WITH_KNOTS('',3,(#14748,#14749,#14750,#14751),
 .UNSPECIFIED.,.F.,.F.,(4,4),(0.33189309985356,0.344890320070497),
 .UNSPECIFIED.);
#612=B_SPLINE_CURVE_WITH_KNOTS('',3,(#14753,#14754,#14755,#14756),
 .UNSPECIFIED.,.F.,.F.,(4,4),(0.272490439993122,0.28518037920845),
 .UNSPECIFIED.);
#613=B_SPLINE_CURVE_WITH_KNOTS('',3,(#14758,#14759,#14760,#14761),
 .UNSPECIFIED.,.F.,.F.,(4,4),(0.21445328866871,0.226856759081898),
 .UNSPECIFIED.);
#614=B_SPLINE_CURVE_WITH_KNOTS('',3,(#14763,#14764,#14765,#14766),
 .UNSPECIFIED.,.F.,.F.,(4,4),(0.157691595007123,0.169827160768426),
 .UNSPECIFIED.);
#615=B_SPLINE_CURVE_WITH_KNOTS('',3,(#14792,#14793,#14794,#14795,#14796,
#14797),.UNSPECIFIED.,.F.,.F.,(4,2,4),(0.,0.510141450492869,1.),
 .UNSPECIFIED.);
#616=B_SPLINE_CURVE_WITH_KNOTS('',3,(#14815,#14816,#14817,#14818),
 .UNSPECIFIED.,.F.,.F.,(4,4),(0.102124791024766,0.114009094135949),
 .UNSPECIFIED.);
#1093=PLANE('',#10131);
#1094=PLANE('',#10132);
#1095=PLANE('',#10133);
#1096=PLANE('',#10134);
#1097=PLANE('',#10135);
#1098=PLANE('',#10136);
#1099=PLANE('',#10137);
#1100=PLANE('',#10138);
#1101=PLANE('',#10139);
#1102=PLANE('',#10140);
#1103=PLANE('',#10141);
#1104=PLANE('',#10142);
#1105=PLANE('',#10143);
#1106=PLANE('',#10144);
#1107=PLANE('',#10145);
#1108=PLANE('',#10146);
#1109=PLANE('',#10147);
#1110=PLANE('',#10148);
#1111=PLANE('',#10149);
#1112=PLANE('',#10150);
#1113=PLANE('',#10151);
#1114=PLANE('',#10152);
#1115=PLANE('',#10153);
#1116=PLANE('',#10154);
#1117=PLANE('',#10155);
#1118=PLANE('',#10156);
#1119=PLANE('',#10157);
#1120=PLANE('',#10158);
#1121=PLANE('',#10159);
#1122=PLANE('',#10160);
#1123=PLANE('',#10161);
#1124=PLANE('',#10162);
#1125=PLANE('',#10163);
#1126=PLANE('',#10164);
#1127=PLANE('',#10165);
#1128=PLANE('',#10166);
#1129=PLANE('',#10167);
#1130=PLANE('',#10168);
#1131=PLANE('',#10169);
#1132=PLANE('',#10170);
#1133=PLANE('',#10171);
#1134=PLANE('',#10172);
#1135=PLANE('',#10173);
#1136=PLANE('',#10174);
#1137=PLANE('',#10175);
#1138=PLANE('',#10176);
#1139=PLANE('',#10177);
#1140=PLANE('',#10178);
#1141=PLANE('',#10179);
#1142=PLANE('',#10180);
#1143=PLANE('',#10181);
#1144=PLANE('',#10182);
#1145=PLANE('',#10183);
#1146=PLANE('',#10184);
#1147=PLANE('',#10185);
#1148=PLANE('',#10186);
#1149=PLANE('',#10187);
#1150=PLANE('',#10188);
#1151=PLANE('',#10189);
#1152=PLANE('',#10190);
#1153=PLANE('',#10191);
#1154=PLANE('',#10192);
#1155=PLANE('',#10193);
#1156=PLANE('',#10194);
#1157=PLANE('',#10195);
#1158=PLANE('',#10196);
#1159=PLANE('',#10197);
#1160=PLANE('',#10198);
#1161=PLANE('',#10199);
#1162=PLANE('',#10200);
#1163=PLANE('',#10201);
#1164=PLANE('',#10202);
#1165=PLANE('',#10203);
#1166=PLANE('',#10204);
#1167=PLANE('',#10205);
#1168=PLANE('',#10206);
#1169=PLANE('',#10207);
#1170=PLANE('',#10208);
#1171=PLANE('',#10209);
#1172=PLANE('',#10210);
#1173=PLANE('',#10211);
#1174=PLANE('',#10212);
#1175=PLANE('',#10213);
#1176=PLANE('',#10214);
#1177=PLANE('',#10215);
#1178=PLANE('',#10216);
#1179=PLANE('',#10223);
#1180=PLANE('',#10224);
#1181=PLANE('',#10225);
#1182=PLANE('',#10226);
#1183=PLANE('',#10227);
#1184=PLANE('',#10228);
#1185=PLANE('',#10229);
#1186=PLANE('',#10230);
#1412=FACE_OUTER_BOUND('',#1971,.T.);
#1413=FACE_OUTER_BOUND('',#1972,.T.);
#1414=FACE_OUTER_BOUND('',#1973,.T.);
#1415=FACE_OUTER_BOUND('',#1974,.T.);
#1416=FACE_OUTER_BOUND('',#1975,.T.);
#1417=FACE_OUTER_BOUND('',#1976,.T.);
#1418=FACE_OUTER_BOUND('',#1977,.T.);
#1419=FACE_OUTER_BOUND('',#1978,.T.);
#1420=FACE_OUTER_BOUND('',#1979,.T.);
#1421=FACE_OUTER_BOUND('',#1980,.T.);
#1422=FACE_OUTER_BOUND('',#1981,.T.);
#1423=FACE_OUTER_BOUND('',#1982,.T.);
#1424=FACE_OUTER_BOUND('',#1983,.T.);
#1425=FACE_OUTER_BOUND('',#1984,.T.);
#1426=FACE_OUTER_BOUND('',#1985,.T.);
#1427=FACE_OUTER_BOUND('',#1986,.T.);
#1428=FACE_OUTER_BOUND('',#1987,.T.);
#1429=FACE_OUTER_BOUND('',#1988,.T.);
#1430=FACE_OUTER_BOUND('',#1989,.T.);
#1431=FACE_OUTER_BOUND('',#1990,.T.);
#1432=FACE_OUTER_BOUND('',#1991,.T.);
#1433=FACE_OUTER_BOUND('',#1992,.T.);
#1434=FACE_OUTER_BOUND('',#1993,.T.);
#1435=FACE_OUTER_BOUND('',#1994,.T.);
#1436=FACE_OUTER_BOUND('',#1995,.T.);
#1437=FACE_OUTER_BOUND('',#1996,.T.);
#1438=FACE_OUTER_BOUND('',#1997,.T.);
#1439=FACE_OUTER_BOUND('',#1998,.T.);
#1440=FACE_OUTER_BOUND('',#1999,.T.);
#1441=FACE_OUTER_BOUND('',#2000,.T.);
#1442=FACE_OUTER_BOUND('',#2001,.T.);
#1443=FACE_OUTER_BOUND('',#2002,.T.);
#1444=FACE_OUTER_BOUND('',#2003,.T.);
#1445=FACE_OUTER_BOUND('',#2004,.T.);
#1446=FACE_OUTER_BOUND('',#2005,.T.);
#1447=FACE_OUTER_BOUND('',#2006,.T.);
#1448=FACE_OUTER_BOUND('',#2007,.T.);
#1449=FACE_OUTER_BOUND('',#2008,.T.);
#1450=FACE_OUTER_BOUND('',#2009,.T.);
#1451=FACE_OUTER_BOUND('',#2010,.T.);
#1452=FACE_OUTER_BOUND('',#2011,.T.);
#1453=FACE_OUTER_BOUND('',#2012,.T.);
#1454=FACE_OUTER_BOUND('',#2013,.T.);
#1455=FACE_OUTER_BOUND('',#2014,.T.);
#1456=FACE_OUTER_BOUND('',#2015,.T.);
#1457=FACE_OUTER_BOUND('',#2016,.T.);
#1458=FACE_OUTER_BOUND('',#2017,.T.);
#1459=FACE_OUTER_BOUND('',#2018,.T.);
#1460=FACE_OUTER_BOUND('',#2019,.T.);
#1461=FACE_OUTER_BOUND('',#2020,.T.);
#1462=FACE_OUTER_BOUND('',#2021,.T.);
#1463=FACE_OUTER_BOUND('',#2022,.T.);
#1464=FACE_OUTER_BOUND('',#2023,.T.);
#1465=FACE_OUTER_BOUND('',#2024,.T.);
#1466=FACE_OUTER_BOUND('',#2025,.T.);
#1467=FACE_OUTER_BOUND('',#2026,.T.);
#1468=FACE_OUTER_BOUND('',#2027,.T.);
#1469=FACE_OUTER_BOUND('',#2028,.T.);
#1470=FACE_OUTER_BOUND('',#2029,.T.);
#1471=FACE_OUTER_BOUND('',#2030,.T.);
#1472=FACE_OUTER_BOUND('',#2031,.T.);
#1473=FACE_OUTER_BOUND('',#2032,.T.);
#1474=FACE_OUTER_BOUND('',#2033,.T.);
#1475=FACE_OUTER_BOUND('',#2034,.T.);
#1476=FACE_OUTER_BOUND('',#2035,.T.);
#1477=FACE_OUTER_BOUND('',#2036,.T.);
#1478=FACE_OUTER_BOUND('',#2037,.T.);
#1479=FACE_OUTER_BOUND('',#2038,.T.);
#1480=FACE_OUTER_BOUND('',#2039,.T.);
#1481=FACE_OUTER_BOUND('',#2040,.T.);
#1482=FACE_OUTER_BOUND('',#2041,.T.);
#1483=FACE_OUTER_BOUND('',#2042,.T.);
#1484=FACE_OUTER_BOUND('',#2043,.T.);
#1485=FACE_OUTER_BOUND('',#2044,.T.);
#1486=FACE_OUTER_BOUND('',#2045,.T.);
#1487=FACE_OUTER_BOUND('',#2046,.T.);
#1488=FACE_OUTER_BOUND('',#2047,.T.);
#1489=FACE_OUTER_BOUND('',#2048,.T.);
#1490=FACE_OUTER_BOUND('',#2049,.T.);
#1491=FACE_OUTER_BOUND('',#2050,.T.);
#1492=FACE_OUTER_BOUND('',#2051,.T.);
#1493=FACE_OUTER_BOUND('',#2052,.T.);
#1494=FACE_OUTER_BOUND('',#2053,.T.);
#1495=FACE_OUTER_BOUND('',#2054,.T.);
#1496=FACE_OUTER_BOUND('',#2055,.T.);
#1497=FACE_OUTER_BOUND('',#2056,.T.);
#1498=FACE_OUTER_BOUND('',#2057,.T.);
#1499=FACE_OUTER_BOUND('',#2058,.T.);
#1500=FACE_OUTER_BOUND('',#2059,.T.);
#1501=FACE_OUTER_BOUND('',#2060,.T.);
#1502=FACE_OUTER_BOUND('',#2061,.T.);
#1503=FACE_OUTER_BOUND('',#2062,.T.);
#1504=FACE_OUTER_BOUND('',#2063,.T.);
#1505=FACE_OUTER_BOUND('',#2064,.T.);
#1506=FACE_OUTER_BOUND('',#2065,.T.);
#1507=FACE_OUTER_BOUND('',#2069,.T.);
#1508=FACE_OUTER_BOUND('',#2070,.T.);
#1509=FACE_OUTER_BOUND('',#2071,.T.);
#1510=FACE_OUTER_BOUND('',#2072,.T.);
#1511=FACE_OUTER_BOUND('',#2073,.T.);
#1512=FACE_OUTER_BOUND('',#2074,.T.);
#1513=FACE_OUTER_BOUND('',#2075,.T.);
#1971=EDGE_LOOP('',(#6853,#6854,#6855,#6856));
#1972=EDGE_LOOP('',(#6857,#6858,#6859,#6860));
#1973=EDGE_LOOP('',(#6861,#6862,#6863,#6864));
#1974=EDGE_LOOP('',(#6865,#6866,#6867,#6868));
#1975=EDGE_LOOP('',(#6869,#6870,#6871,#6872));
#1976=EDGE_LOOP('',(#6873,#6874,#6875,#6876));
#1977=EDGE_LOOP('',(#6877,#6878,#6879,#6880));
#1978=EDGE_LOOP('',(#6881,#6882,#6883,#6884));
#1979=EDGE_LOOP('',(#6885,#6886,#6887,#6888));
#1980=EDGE_LOOP('',(#6889,#6890,#6891,#6892));
#1981=EDGE_LOOP('',(#6893,#6894,#6895,#6896));
#1982=EDGE_LOOP('',(#6897,#6898,#6899,#6900));
#1983=EDGE_LOOP('',(#6901,#6902,#6903,#6904));
#1984=EDGE_LOOP('',(#6905,#6906,#6907,#6908));
#1985=EDGE_LOOP('',(#6909,#6910,#6911,#6912));
#1986=EDGE_LOOP('',(#6913,#6914,#6915,#6916));
#1987=EDGE_LOOP('',(#6917,#6918,#6919,#6920));
#1988=EDGE_LOOP('',(#6921,#6922,#6923,#6924));
#1989=EDGE_LOOP('',(#6925,#6926,#6927,#6928));
#1990=EDGE_LOOP('',(#6929,#6930,#6931,#6932));
#1991=EDGE_LOOP('',(#6933,#6934,#6935,#6936));
#1992=EDGE_LOOP('',(#6937,#6938,#6939,#6940));
#1993=EDGE_LOOP('',(#6941,#6942,#6943,#6944));
#1994=EDGE_LOOP('',(#6945,#6946,#6947,#6948));
#1995=EDGE_LOOP('',(#6949,#6950,#6951,#6952));
#1996=EDGE_LOOP('',(#6953,#6954,#6955,#6956));
#1997=EDGE_LOOP('',(#6957,#6958,#6959,#6960));
#1998=EDGE_LOOP('',(#6961,#6962,#6963,#6964));
#1999=EDGE_LOOP('',(#6965,#6966,#6967,#6968));
#2000=EDGE_LOOP('',(#6969,#6970,#6971,#6972));
#2001=EDGE_LOOP('',(#6973,#6974,#6975,#6976));
#2002=EDGE_LOOP('',(#6977,#6978,#6979,#6980));
#2003=EDGE_LOOP('',(#6981,#6982,#6983,#6984));
#2004=EDGE_LOOP('',(#6985,#6986,#6987,#6988));
#2005=EDGE_LOOP('',(#6989,#6990,#6991,#6992));
#2006=EDGE_LOOP('',(#6993,#6994,#6995,#6996));
#2007=EDGE_LOOP('',(#6997,#6998,#6999,#7000));
#2008=EDGE_LOOP('',(#7001,#7002,#7003,#7004));
#2009=EDGE_LOOP('',(#7005,#7006,#7007,#7008));
#2010=EDGE_LOOP('',(#7009,#7010,#7011,#7012));
#2011=EDGE_LOOP('',(#7013,#7014,#7015,#7016));
#2012=EDGE_LOOP('',(#7017,#7018,#7019,#7020));
#2013=EDGE_LOOP('',(#7021,#7022,#7023,#7024));
#2014=EDGE_LOOP('',(#7025,#7026,#7027,#7028));
#2015=EDGE_LOOP('',(#7029,#7030,#7031,#7032));
#2016=EDGE_LOOP('',(#7033,#7034,#7035,#7036));
#2017=EDGE_LOOP('',(#7037,#7038,#7039,#7040));
#2018=EDGE_LOOP('',(#7041,#7042,#7043,#7044));
#2019=EDGE_LOOP('',(#7045,#7046,#7047,#7048));
#2020=EDGE_LOOP('',(#7049,#7050,#7051,#7052));
#2021=EDGE_LOOP('',(#7053,#7054,#7055,#7056));
#2022=EDGE_LOOP('',(#7057,#7058,#7059,#7060));
#2023=EDGE_LOOP('',(#7061,#7062,#7063,#7064));
#2024=EDGE_LOOP('',(#7065,#7066,#7067,#7068));
#2025=EDGE_LOOP('',(#7069,#7070,#7071,#7072));
#2026=EDGE_LOOP('',(#7073,#7074,#7075,#7076));
#2027=EDGE_LOOP('',(#7077,#7078,#7079,#7080));
#2028=EDGE_LOOP('',(#7081,#7082,#7083,#7084,#7085,#7086,#7087,#7088,#7089,
#7090,#7091,#7092,#7093,#7094,#7095,#7096,#7097,#7098,#7099,#7100,#7101,
#7102,#7103,#7104,#7105,#7106,#7107,#7108,#7109,#7110,#7111,#7112,#7113,
#7114,#7115,#7116,#7117,#7118,#7119,#7120,#7121,#7122,#7123,#7124,#7125,
#7126,#7127,#7128,#7129,#7130,#7131,#7132,#7133,#7134,#7135,#7136,#7137,
#7138,#7139,#7140,#7141,#7142,#7143,#7144,#7145,#7146,#7147,#7148,#7149,
#7150,#7151,#7152,#7153,#7154,#7155,#7156,#7157,#7158,#7159,#7160,#7161,
#7162,#7163,#7164,#7165));
#2029=EDGE_LOOP('',(#7166,#7167,#7168,#7169));
#2030=EDGE_LOOP('',(#7170,#7171,#7172,#7173,#7174,#7175,#7176));
#2031=EDGE_LOOP('',(#7177,#7178,#7179,#7180));
#2032=EDGE_LOOP('',(#7181,#7182,#7183,#7184));
#2033=EDGE_LOOP('',(#7185,#7186,#7187,#7188));
#2034=EDGE_LOOP('',(#7189,#7190,#7191,#7192));
#2035=EDGE_LOOP('',(#7193,#7194,#7195,#7196));
#2036=EDGE_LOOP('',(#7197,#7198,#7199,#7200));
#2037=EDGE_LOOP('',(#7201,#7202,#7203,#7204));
#2038=EDGE_LOOP('',(#7205,#7206,#7207,#7208));
#2039=EDGE_LOOP('',(#7209,#7210,#7211,#7212));
#2040=EDGE_LOOP('',(#7213,#7214,#7215,#7216));
#2041=EDGE_LOOP('',(#7217,#7218,#7219,#7220));
#2042=EDGE_LOOP('',(#7221,#7222,#7223,#7224));
#2043=EDGE_LOOP('',(#7225,#7226,#7227,#7228));
#2044=EDGE_LOOP('',(#7229,#7230,#7231,#7232));
#2045=EDGE_LOOP('',(#7233,#7234,#7235,#7236));
#2046=EDGE_LOOP('',(#7237,#7238,#7239,#7240));
#2047=EDGE_LOOP('',(#7241,#7242,#7243,#7244));
#2048=EDGE_LOOP('',(#7245,#7246,#7247,#7248));
#2049=EDGE_LOOP('',(#7249,#7250,#7251,#7252));
#2050=EDGE_LOOP('',(#7253,#7254,#7255,#7256));
#2051=EDGE_LOOP('',(#7257,#7258,#7259,#7260));
#2052=EDGE_LOOP('',(#7261,#7262,#7263,#7264));
#2053=EDGE_LOOP('',(#7265,#7266,#7267,#7268));
#2054=EDGE_LOOP('',(#7269,#7270,#7271,#7272));
#2055=EDGE_LOOP('',(#7273,#7274,#7275,#7276));
#2056=EDGE_LOOP('',(#7277,#7278,#7279,#7280));
#2057=EDGE_LOOP('',(#7281,#7282,#7283,#7284));
#2058=EDGE_LOOP('',(#7285,#7286,#7287,#7288,#7289));
#2059=EDGE_LOOP('',(#7290,#7291,#7292,#7293,#7294,#7295,#7296,#7297,#7298,
#7299,#7300,#7301,#7302,#7303,#7304,#7305,#7306,#7307,#7308,#7309,#7310,
#7311,#7312,#7313,#7314,#7315,#7316,#7317,#7318,#7319,#7320,#7321,#7322,
#7323,#7324,#7325,#7326,#7327,#7328,#7329,#7330,#7331,#7332,#7333,#7334,
#7335,#7336,#7337,#7338,#7339,#7340,#7341,#7342,#7343,#7344,#7345,#7346,
#7347,#7348,#7349,#7350,#7351,#7352,#7353,#7354,#7355,#7356,#7357,#7358,
#7359,#7360,#7361,#7362,#7363,#7364,#7365,#7366,#7367,#7368,#7369,#7370,
#7371,#7372,#7373,#7374));
#2060=EDGE_LOOP('',(#7375,#7376,#7377,#7378));
#2061=EDGE_LOOP('',(#7379,#7380,#7381,#7382));
#2062=EDGE_LOOP('',(#7383,#7384,#7385,#7386));
#2063=EDGE_LOOP('',(#7387,#7388,#7389,#7390));
#2064=EDGE_LOOP('',(#7391,#7392,#7393,#7394));
#2065=EDGE_LOOP('',(#7395,#7396,#7397,#7398,#7399,#7400,#7401,#7402,#7403,
#7404,#7405,#7406));
#2066=EDGE_LOOP('',(#7407));
#2067=EDGE_LOOP('',(#7408));
#2068=EDGE_LOOP('',(#7409));
#2069=EDGE_LOOP('',(#7410,#7411,#7412,#7413));
#2070=EDGE_LOOP('',(#7414,#7415,#7416,#7417));
#2071=EDGE_LOOP('',(#7418,#7419,#7420,#7421));
#2072=EDGE_LOOP('',(#7422,#7423,#7424,#7425));
#2073=EDGE_LOOP('',(#7426,#7427,#7428,#7429));
#2074=EDGE_LOOP('',(#7430,#7431,#7432,#7433));
#2075=EDGE_LOOP('',(#7434,#7435,#7436,#7437,#7438,#7439,#7440,#7441,#7442,
#7443,#7444,#7445));
#2076=EDGE_LOOP('',(#7446));
#2077=EDGE_LOOP('',(#7447));
#2078=EDGE_LOOP('',(#7448));
#2605=LINE('',#13739,#3193);
#2606=LINE('',#13745,#3194);
#2607=LINE('',#13751,#3195);
#2608=LINE('',#13761,#3196);
#2609=LINE('',#13767,#3197);
#2610=LINE('',#13775,#3198);
#2611=LINE('',#13788,#3199);
#2612=LINE('',#13794,#3200);
#2613=LINE('',#13802,#3201);
#2614=LINE('',#13815,#3202);
#2615=LINE('',#13821,#3203);
#2616=LINE('',#13829,#3204);
#2617=LINE('',#13842,#3205);
#2618=LINE('',#13848,#3206);
#2619=LINE('',#13856,#3207);
#2620=LINE('',#13869,#3208);
#2621=LINE('',#13875,#3209);
#2622=LINE('',#13883,#3210);
#2623=LINE('',#13896,#3211);
#2624=LINE('',#13902,#3212);
#2625=LINE('',#13910,#3213);
#2626=LINE('',#13923,#3214);
#2627=LINE('',#13929,#3215);
#2628=LINE('',#13937,#3216);
#2629=LINE('',#13950,#3217);
#2630=LINE('',#13956,#3218);
#2631=LINE('',#13964,#3219);
#2632=LINE('',#13977,#3220);
#2633=LINE('',#13983,#3221);
#2634=LINE('',#13991,#3222);
#2635=LINE('',#14004,#3223);
#2636=LINE('',#14010,#3224);
#2637=LINE('',#14018,#3225);
#2638=LINE('',#14031,#3226);
#2639=LINE('',#14037,#3227);
#2640=LINE('',#14045,#3228);
#2641=LINE('',#14058,#3229);
#2642=LINE('',#14064,#3230);
#2643=LINE('',#14072,#3231);
#2644=LINE('',#14085,#3232);
#2645=LINE('',#14091,#3233);
#2646=LINE('',#14099,#3234);
#2647=LINE('',#14112,#3235);
#2648=LINE('',#14118,#3236);
#2649=LINE('',#14126,#3237);
#2650=LINE('',#14139,#3238);
#2651=LINE('',#14145,#3239);
#2652=LINE('',#14153,#3240);
#2653=LINE('',#14166,#3241);
#2654=LINE('',#14172,#3242);
#2655=LINE('',#14180,#3243);
#2656=LINE('',#14193,#3244);
#2657=LINE('',#14199,#3245);
#2658=LINE('',#14207,#3246);
#2659=LINE('',#14220,#3247);
#2660=LINE('',#14226,#3248);
#2661=LINE('',#14234,#3249);
#2662=LINE('',#14247,#3250);
#2663=LINE('',#14253,#3251);
#2664=LINE('',#14261,#3252);
#2665=LINE('',#14274,#3253);
#2666=LINE('',#14280,#3254);
#2667=LINE('',#14288,#3255);
#2668=LINE('',#14301,#3256);
#2669=LINE('',#14307,#3257);
#2670=LINE('',#14315,#3258);
#2671=LINE('',#14328,#3259);
#2672=LINE('',#14334,#3260);
#2673=LINE('',#14342,#3261);
#2674=LINE('',#14355,#3262);
#2675=LINE('',#14361,#3263);
#2676=LINE('',#14369,#3264);
#2677=LINE('',#14382,#3265);
#2678=LINE('',#14388,#3266);
#2679=LINE('',#14396,#3267);
#2680=LINE('',#14409,#3268);
#2681=LINE('',#14415,#3269);
#2682=LINE('',#14423,#3270);
#2683=LINE('',#14436,#3271);
#2684=LINE('',#14442,#3272);
#2685=LINE('',#14450,#3273);
#2686=LINE('',#14463,#3274);
#2687=LINE('',#14469,#3275);
#2688=LINE('',#14477,#3276);
#2689=LINE('',#14604,#3277);
#2690=LINE('',#14613,#3278);
#2691=LINE('',#14628,#3279);
#2692=LINE('',#14631,#3280);
#2693=LINE('',#14633,#3281);
#2694=LINE('',#14635,#3282);
#2695=LINE('',#14637,#3283);
#2696=LINE('',#14769,#3284);
#2697=LINE('',#14770,#3285);
#2698=LINE('',#14773,#3286);
#2699=LINE('',#14774,#3287);
#2700=LINE('',#14798,#3288);
#2701=LINE('',#14819,#3289);
#2702=LINE('',#14823,#3290);
#2703=LINE('',#14825,#3291);
#2704=LINE('',#14826,#3292);
#2705=LINE('',#14830,#3293);
#2706=LINE('',#14831,#3294);
#2707=LINE('',#14832,#3295);
#2708=LINE('',#14837,#3296);
#2709=LINE('',#14843,#3297);
#2710=LINE('',#14847,#3298);
#2711=LINE('',#14849,#3299);
#2712=LINE('',#14851,#3300);
#2713=LINE('',#14853,#3301);
#2714=LINE('',#14855,#3302);
#2715=LINE('',#14856,#3303);
#2716=LINE('',#14859,#3304);
#2717=LINE('',#14860,#3305);
#2718=LINE('',#14863,#3306);
#2719=LINE('',#14864,#3307);
#2720=LINE('',#14867,#3308);
#2721=LINE('',#14868,#3309);
#2722=LINE('',#14871,#3310);
#2723=LINE('',#14872,#3311);
#2724=LINE('',#14875,#3312);
#2725=LINE('',#14876,#3313);
#2726=LINE('',#14878,#3314);
#3193=VECTOR('',#11023,0.17);
#3194=VECTOR('',#11030,0.17);
#3195=VECTOR('',#11037,0.41);
#3196=VECTOR('',#11042,1.);
#3197=VECTOR('',#11043,1.);
#3198=VECTOR('',#11046,1.);
#3199=VECTOR('',#11049,1.);
#3200=VECTOR('',#11050,1.);
#3201=VECTOR('',#11053,1.);
#3202=VECTOR('',#11056,1.);
#3203=VECTOR('',#11057,1.);
#3204=VECTOR('',#11060,1.);
#3205=VECTOR('',#11063,1.);
#3206=VECTOR('',#11064,1.);
#3207=VECTOR('',#11067,1.);
#3208=VECTOR('',#11070,1.);
#3209=VECTOR('',#11071,1.);
#3210=VECTOR('',#11074,1.);
#3211=VECTOR('',#11077,1.);
#3212=VECTOR('',#11078,1.);
#3213=VECTOR('',#11081,1.);
#3214=VECTOR('',#11084,1.);
#3215=VECTOR('',#11085,1.);
#3216=VECTOR('',#11088,1.);
#3217=VECTOR('',#11091,1.);
#3218=VECTOR('',#11092,1.);
#3219=VECTOR('',#11095,1.);
#3220=VECTOR('',#11098,1.);
#3221=VECTOR('',#11099,1.);
#3222=VECTOR('',#11102,1.);
#3223=VECTOR('',#11105,1.);
#3224=VECTOR('',#11106,1.);
#3225=VECTOR('',#11109,1.);
#3226=VECTOR('',#11112,1.);
#3227=VECTOR('',#11113,1.);
#3228=VECTOR('',#11116,1.);
#3229=VECTOR('',#11119,1.);
#3230=VECTOR('',#11120,1.);
#3231=VECTOR('',#11123,1.);
#3232=VECTOR('',#11126,1.);
#3233=VECTOR('',#11127,1.);
#3234=VECTOR('',#11130,1.);
#3235=VECTOR('',#11133,1.);
#3236=VECTOR('',#11134,1.);
#3237=VECTOR('',#11137,1.);
#3238=VECTOR('',#11140,1.);
#3239=VECTOR('',#11141,1.);
#3240=VECTOR('',#11144,1.);
#3241=VECTOR('',#11147,1.);
#3242=VECTOR('',#11148,1.);
#3243=VECTOR('',#11151,1.);
#3244=VECTOR('',#11154,1.);
#3245=VECTOR('',#11155,1.);
#3246=VECTOR('',#11158,1.);
#3247=VECTOR('',#11161,1.);
#3248=VECTOR('',#11162,1.);
#3249=VECTOR('',#11165,1.);
#3250=VECTOR('',#11168,1.);
#3251=VECTOR('',#11169,1.);
#3252=VECTOR('',#11172,1.);
#3253=VECTOR('',#11175,1.);
#3254=VECTOR('',#11176,1.);
#3255=VECTOR('',#11179,1.);
#3256=VECTOR('',#11182,1.);
#3257=VECTOR('',#11183,1.);
#3258=VECTOR('',#11186,1.);
#3259=VECTOR('',#11189,1.);
#3260=VECTOR('',#11190,1.);
#3261=VECTOR('',#11193,1.);
#3262=VECTOR('',#11196,1.);
#3263=VECTOR('',#11197,1.);
#3264=VECTOR('',#11200,1.);
#3265=VECTOR('',#11203,1.);
#3266=VECTOR('',#11204,1.);
#3267=VECTOR('',#11207,1.);
#3268=VECTOR('',#11210,1.);
#3269=VECTOR('',#11211,1.);
#3270=VECTOR('',#11214,1.);
#3271=VECTOR('',#11217,1.);
#3272=VECTOR('',#11218,1.);
#3273=VECTOR('',#11221,1.);
#3274=VECTOR('',#11224,1.);
#3275=VECTOR('',#11225,1.);
#3276=VECTOR('',#11228,1.);
#3277=VECTOR('',#11229,1.);
#3278=VECTOR('',#11230,1.);
#3279=VECTOR('',#11233,1.);
#3280=VECTOR('',#11236,1.);
#3281=VECTOR('',#11237,1.);
#3282=VECTOR('',#11238,1.);
#3283=VECTOR('',#11239,1.);
#3284=VECTOR('',#11292,1.);
#3285=VECTOR('',#11293,1.);
#3286=VECTOR('',#11296,1.);
#3287=VECTOR('',#11297,1.);
#3288=VECTOR('',#11298,1.);
#3289=VECTOR('',#11299,1.);
#3290=VECTOR('',#11304,1.);
#3291=VECTOR('',#11305,1.);
#3292=VECTOR('',#11306,1.);
#3293=VECTOR('',#11309,1.);
#3294=VECTOR('',#11310,1.);
#3295=VECTOR('',#11311,1.);
#3296=VECTOR('',#11316,1.);
#3297=VECTOR('',#11323,1.);
#3298=VECTOR('',#11328,1.);
#3299=VECTOR('',#11329,1.);
#3300=VECTOR('',#11330,1.);
#3301=VECTOR('',#11331,1.);
#3302=VECTOR('',#11332,1.);
#3303=VECTOR('',#11333,1.);
#3304=VECTOR('',#11336,1.);
#3305=VECTOR('',#11337,1.);
#3306=VECTOR('',#11340,1.);
#3307=VECTOR('',#11341,1.);
#3308=VECTOR('',#11344,1.);
#3309=VECTOR('',#11345,1.);
#3310=VECTOR('',#11348,1.);
#3311=VECTOR('',#11349,1.);
#3312=VECTOR('',#11352,1.);
#3313=VECTOR('',#11353,1.);
#3314=VECTOR('',#11356,1.);
#3669=CIRCLE('',#10123,0.17);
#3670=CIRCLE('',#10124,0.17);
#3671=CIRCLE('',#10126,0.17);
#3672=CIRCLE('',#10127,0.17);
#3673=CIRCLE('',#10129,0.41);
#3674=CIRCLE('',#10130,0.41);
#3675=CIRCLE('',#10218,1.4);
#3676=CIRCLE('',#10219,1.4);
#3677=CIRCLE('',#10221,1.4);
#3678=CIRCLE('',#10222,1.4);
#4025=VERTEX_POINT('',#13736);
#4026=VERTEX_POINT('',#13738);
#4027=VERTEX_POINT('',#13742);
#4028=VERTEX_POINT('',#13744);
#4029=VERTEX_POINT('',#13748);
#4030=VERTEX_POINT('',#13750);
#4031=VERTEX_POINT('',#13754);
#4032=VERTEX_POINT('',#13755);
#4033=VERTEX_POINT('',#13760);
#4034=VERTEX_POINT('',#13762);
#4035=VERTEX_POINT('',#13769);
#4036=VERTEX_POINT('',#13774);
#4037=VERTEX_POINT('',#13781);
#4038=VERTEX_POINT('',#13782);
#4039=VERTEX_POINT('',#13787);
#4040=VERTEX_POINT('',#13789);
#4041=VERTEX_POINT('',#13796);
#4042=VERTEX_POINT('',#13801);
#4043=VERTEX_POINT('',#13808);
#4044=VERTEX_POINT('',#13809);
#4045=VERTEX_POINT('',#13814);
#4046=VERTEX_POINT('',#13816);
#4047=VERTEX_POINT('',#13823);
#4048=VERTEX_POINT('',#13828);
#4049=VERTEX_POINT('',#13835);
#4050=VERTEX_POINT('',#13836);
#4051=VERTEX_POINT('',#13841);
#4052=VERTEX_POINT('',#13843);
#4053=VERTEX_POINT('',#13850);
#4054=VERTEX_POINT('',#13855);
#4055=VERTEX_POINT('',#13862);
#4056=VERTEX_POINT('',#13863);
#4057=VERTEX_POINT('',#13868);
#4058=VERTEX_POINT('',#13870);
#4059=VERTEX_POINT('',#13877);
#4060=VERTEX_POINT('',#13882);
#4061=VERTEX_POINT('',#13889);
#4062=VERTEX_POINT('',#13890);
#4063=VERTEX_POINT('',#13895);
#4064=VERTEX_POINT('',#13897);
#4065=VERTEX_POINT('',#13904);
#4066=VERTEX_POINT('',#13909);
#4067=VERTEX_POINT('',#13916);
#4068=VERTEX_POINT('',#13917);
#4069=VERTEX_POINT('',#13922);
#4070=VERTEX_POINT('',#13924);
#4071=VERTEX_POINT('',#13931);
#4072=VERTEX_POINT('',#13936);
#4073=VERTEX_POINT('',#13943);
#4074=VERTEX_POINT('',#13944);
#4075=VERTEX_POINT('',#13949);
#4076=VERTEX_POINT('',#13951);
#4077=VERTEX_POINT('',#13958);
#4078=VERTEX_POINT('',#13963);
#4079=VERTEX_POINT('',#13970);
#4080=VERTEX_POINT('',#13971);
#4081=VERTEX_POINT('',#13976);
#4082=VERTEX_POINT('',#13978);
#4083=VERTEX_POINT('',#13985);
#4084=VERTEX_POINT('',#13990);
#4085=VERTEX_POINT('',#13997);
#4086=VERTEX_POINT('',#13998);
#4087=VERTEX_POINT('',#14003);
#4088=VERTEX_POINT('',#14005);
#4089=VERTEX_POINT('',#14012);
#4090=VERTEX_POINT('',#14017);
#4091=VERTEX_POINT('',#14024);
#4092=VERTEX_POINT('',#14025);
#4093=VERTEX_POINT('',#14030);
#4094=VERTEX_POINT('',#14032);
#4095=VERTEX_POINT('',#14039);
#4096=VERTEX_POINT('',#14044);
#4097=VERTEX_POINT('',#14051);
#4098=VERTEX_POINT('',#14052);
#4099=VERTEX_POINT('',#14057);
#4100=VERTEX_POINT('',#14059);
#4101=VERTEX_POINT('',#14066);
#4102=VERTEX_POINT('',#14071);
#4103=VERTEX_POINT('',#14078);
#4104=VERTEX_POINT('',#14079);
#4105=VERTEX_POINT('',#14084);
#4106=VERTEX_POINT('',#14086);
#4107=VERTEX_POINT('',#14093);
#4108=VERTEX_POINT('',#14098);
#4109=VERTEX_POINT('',#14105);
#4110=VERTEX_POINT('',#14106);
#4111=VERTEX_POINT('',#14111);
#4112=VERTEX_POINT('',#14113);
#4113=VERTEX_POINT('',#14120);
#4114=VERTEX_POINT('',#14125);
#4115=VERTEX_POINT('',#14132);
#4116=VERTEX_POINT('',#14133);
#4117=VERTEX_POINT('',#14138);
#4118=VERTEX_POINT('',#14140);
#4119=VERTEX_POINT('',#14147);
#4120=VERTEX_POINT('',#14152);
#4121=VERTEX_POINT('',#14159);
#4122=VERTEX_POINT('',#14160);
#4123=VERTEX_POINT('',#14165);
#4124=VERTEX_POINT('',#14167);
#4125=VERTEX_POINT('',#14174);
#4126=VERTEX_POINT('',#14179);
#4127=VERTEX_POINT('',#14186);
#4128=VERTEX_POINT('',#14187);
#4129=VERTEX_POINT('',#14192);
#4130=VERTEX_POINT('',#14194);
#4131=VERTEX_POINT('',#14201);
#4132=VERTEX_POINT('',#14206);
#4133=VERTEX_POINT('',#14213);
#4134=VERTEX_POINT('',#14214);
#4135=VERTEX_POINT('',#14219);
#4136=VERTEX_POINT('',#14221);
#4137=VERTEX_POINT('',#14228);
#4138=VERTEX_POINT('',#14233);
#4139=VERTEX_POINT('',#14240);
#4140=VERTEX_POINT('',#14241);
#4141=VERTEX_POINT('',#14246);
#4142=VERTEX_POINT('',#14248);
#4143=VERTEX_POINT('',#14255);
#4144=VERTEX_POINT('',#14260);
#4145=VERTEX_POINT('',#14267);
#4146=VERTEX_POINT('',#14268);
#4147=VERTEX_POINT('',#14273);
#4148=VERTEX_POINT('',#14275);
#4149=VERTEX_POINT('',#14282);
#4150=VERTEX_POINT('',#14287);
#4151=VERTEX_POINT('',#14294);
#4152=VERTEX_POINT('',#14295);
#4153=VERTEX_POINT('',#14300);
#4154=VERTEX_POINT('',#14302);
#4155=VERTEX_POINT('',#14309);
#4156=VERTEX_POINT('',#14314);
#4157=VERTEX_POINT('',#14321);
#4158=VERTEX_POINT('',#14322);
#4159=VERTEX_POINT('',#14327);
#4160=VERTEX_POINT('',#14329);
#4161=VERTEX_POINT('',#14336);
#4162=VERTEX_POINT('',#14341);
#4163=VERTEX_POINT('',#14348);
#4164=VERTEX_POINT('',#14349);
#4165=VERTEX_POINT('',#14354);
#4166=VERTEX_POINT('',#14356);
#4167=VERTEX_POINT('',#14363);
#4168=VERTEX_POINT('',#14368);
#4169=VERTEX_POINT('',#14375);
#4170=VERTEX_POINT('',#14376);
#4171=VERTEX_POINT('',#14381);
#4172=VERTEX_POINT('',#14383);
#4173=VERTEX_POINT('',#14390);
#4174=VERTEX_POINT('',#14395);
#4175=VERTEX_POINT('',#14402);
#4176=VERTEX_POINT('',#14403);
#4177=VERTEX_POINT('',#14408);
#4178=VERTEX_POINT('',#14410);
#4179=VERTEX_POINT('',#14417);
#4180=VERTEX_POINT('',#14422);
#4181=VERTEX_POINT('',#14429);
#4182=VERTEX_POINT('',#14430);
#4183=VERTEX_POINT('',#14435);
#4184=VERTEX_POINT('',#14437);
#4185=VERTEX_POINT('',#14444);
#4186=VERTEX_POINT('',#14449);
#4187=VERTEX_POINT('',#14456);
#4188=VERTEX_POINT('',#14457);
#4189=VERTEX_POINT('',#14462);
#4190=VERTEX_POINT('',#14464);
#4191=VERTEX_POINT('',#14471);
#4192=VERTEX_POINT('',#14476);
#4193=VERTEX_POINT('',#14598);
#4194=VERTEX_POINT('',#14603);
#4195=VERTEX_POINT('',#14605);
#4196=VERTEX_POINT('',#14612);
#4197=VERTEX_POINT('',#14623);
#4198=VERTEX_POINT('',#14630);
#4199=VERTEX_POINT('',#14632);
#4200=VERTEX_POINT('',#14634);
#4201=VERTEX_POINT('',#14636);
#4202=VERTEX_POINT('',#14768);
#4203=VERTEX_POINT('',#14772);
#4204=VERTEX_POINT('',#14791);
#4205=VERTEX_POINT('',#14822);
#4206=VERTEX_POINT('',#14824);
#4207=VERTEX_POINT('',#14828);
#4208=VERTEX_POINT('',#14829);
#4209=VERTEX_POINT('',#14834);
#4210=VERTEX_POINT('',#14836);
#4211=VERTEX_POINT('',#14840);
#4212=VERTEX_POINT('',#14842);
#4213=VERTEX_POINT('',#14846);
#4214=VERTEX_POINT('',#14848);
#4215=VERTEX_POINT('',#14850);
#4216=VERTEX_POINT('',#14852);
#4217=VERTEX_POINT('',#14854);
#4218=VERTEX_POINT('',#14858);
#4219=VERTEX_POINT('',#14862);
#4220=VERTEX_POINT('',#14866);
#4221=VERTEX_POINT('',#14870);
#4222=VERTEX_POINT('',#14874);
#5085=EDGE_CURVE('',#4025,#4025,#3669,.T.);
#5086=EDGE_CURVE('',#4025,#4026,#2605,.T.);
#5087=EDGE_CURVE('',#4026,#4026,#3670,.T.);
#5088=EDGE_CURVE('',#4027,#4027,#3671,.T.);
#5089=EDGE_CURVE('',#4027,#4028,#2606,.T.);
#5090=EDGE_CURVE('',#4028,#4028,#3672,.T.);
#5091=EDGE_CURVE('',#4029,#4029,#3673,.T.);
#5092=EDGE_CURVE('',#4029,#4030,#2607,.T.);
#5093=EDGE_CURVE('',#4030,#4030,#3674,.T.);
#5094=EDGE_CURVE('',#4031,#4032,#451,.T.);
#5095=EDGE_CURVE('',#4033,#4031,#2608,.T.);
#5096=EDGE_CURVE('',#4034,#4033,#452,.T.);
#5097=EDGE_CURVE('',#4032,#4034,#2609,.T.);
#5098=EDGE_CURVE('',#4035,#4031,#453,.T.);
#5099=EDGE_CURVE('',#4036,#4035,#2610,.T.);
#5100=EDGE_CURVE('',#4033,#4036,#454,.T.);
#5101=EDGE_CURVE('',#4037,#4038,#455,.T.);
#5102=EDGE_CURVE('',#4039,#4037,#2611,.T.);
#5103=EDGE_CURVE('',#4040,#4039,#456,.T.);
#5104=EDGE_CURVE('',#4038,#4040,#2612,.T.);
#5105=EDGE_CURVE('',#4041,#4037,#457,.T.);
#5106=EDGE_CURVE('',#4042,#4041,#2613,.T.);
#5107=EDGE_CURVE('',#4039,#4042,#458,.T.);
#5108=EDGE_CURVE('',#4043,#4044,#459,.T.);
#5109=EDGE_CURVE('',#4045,#4043,#2614,.T.);
#5110=EDGE_CURVE('',#4046,#4045,#460,.T.);
#5111=EDGE_CURVE('',#4044,#4046,#2615,.T.);
#5112=EDGE_CURVE('',#4047,#4043,#461,.T.);
#5113=EDGE_CURVE('',#4048,#4047,#2616,.T.);
#5114=EDGE_CURVE('',#4045,#4048,#462,.T.);
#5115=EDGE_CURVE('',#4049,#4050,#463,.T.);
#5116=EDGE_CURVE('',#4051,#4049,#2617,.T.);
#5117=EDGE_CURVE('',#4052,#4051,#464,.T.);
#5118=EDGE_CURVE('',#4050,#4052,#2618,.T.);
#5119=EDGE_CURVE('',#4053,#4049,#465,.T.);
#5120=EDGE_CURVE('',#4054,#4053,#2619,.T.);
#5121=EDGE_CURVE('',#4051,#4054,#466,.T.);
#5122=EDGE_CURVE('',#4055,#4056,#467,.T.);
#5123=EDGE_CURVE('',#4057,#4055,#2620,.T.);
#5124=EDGE_CURVE('',#4058,#4057,#468,.T.);
#5125=EDGE_CURVE('',#4056,#4058,#2621,.T.);
#5126=EDGE_CURVE('',#4059,#4055,#469,.T.);
#5127=EDGE_CURVE('',#4060,#4059,#2622,.T.);
#5128=EDGE_CURVE('',#4057,#4060,#470,.T.);
#5129=EDGE_CURVE('',#4061,#4062,#471,.T.);
#5130=EDGE_CURVE('',#4063,#4061,#2623,.T.);
#5131=EDGE_CURVE('',#4064,#4063,#472,.T.);
#5132=EDGE_CURVE('',#4062,#4064,#2624,.T.);
#5133=EDGE_CURVE('',#4065,#4061,#473,.T.);
#5134=EDGE_CURVE('',#4066,#4065,#2625,.T.);
#5135=EDGE_CURVE('',#4063,#4066,#474,.T.);
#5136=EDGE_CURVE('',#4067,#4068,#475,.T.);
#5137=EDGE_CURVE('',#4069,#4067,#2626,.T.);
#5138=EDGE_CURVE('',#4070,#4069,#476,.T.);
#5139=EDGE_CURVE('',#4068,#4070,#2627,.T.);
#5140=EDGE_CURVE('',#4071,#4067,#477,.T.);
#5141=EDGE_CURVE('',#4072,#4071,#2628,.T.);
#5142=EDGE_CURVE('',#4069,#4072,#478,.T.);
#5143=EDGE_CURVE('',#4073,#4074,#479,.T.);
#5144=EDGE_CURVE('',#4075,#4073,#2629,.T.);
#5145=EDGE_CURVE('',#4076,#4075,#480,.T.);
#5146=EDGE_CURVE('',#4074,#4076,#2630,.T.);
#5147=EDGE_CURVE('',#4077,#4073,#481,.T.);
#5148=EDGE_CURVE('',#4078,#4077,#2631,.T.);
#5149=EDGE_CURVE('',#4075,#4078,#482,.T.);
#5150=EDGE_CURVE('',#4079,#4080,#483,.T.);
#5151=EDGE_CURVE('',#4081,#4079,#2632,.T.);
#5152=EDGE_CURVE('',#4082,#4081,#484,.T.);
#5153=EDGE_CURVE('',#4080,#4082,#2633,.T.);
#5154=EDGE_CURVE('',#4083,#4079,#485,.T.);
#5155=EDGE_CURVE('',#4084,#4083,#2634,.T.);
#5156=EDGE_CURVE('',#4081,#4084,#486,.T.);
#5157=EDGE_CURVE('',#4085,#4086,#487,.T.);
#5158=EDGE_CURVE('',#4087,#4085,#2635,.T.);
#5159=EDGE_CURVE('',#4088,#4087,#488,.T.);
#5160=EDGE_CURVE('',#4086,#4088,#2636,.T.);
#5161=EDGE_CURVE('',#4089,#4085,#489,.T.);
#5162=EDGE_CURVE('',#4090,#4089,#2637,.T.);
#5163=EDGE_CURVE('',#4087,#4090,#490,.T.);
#5164=EDGE_CURVE('',#4091,#4092,#491,.T.);
#5165=EDGE_CURVE('',#4093,#4091,#2638,.T.);
#5166=EDGE_CURVE('',#4094,#4093,#492,.T.);
#5167=EDGE_CURVE('',#4092,#4094,#2639,.T.);
#5168=EDGE_CURVE('',#4095,#4091,#493,.T.);
#5169=EDGE_CURVE('',#4096,#4095,#2640,.T.);
#5170=EDGE_CURVE('',#4093,#4096,#494,.T.);
#5171=EDGE_CURVE('',#4097,#4098,#495,.T.);
#5172=EDGE_CURVE('',#4099,#4097,#2641,.T.);
#5173=EDGE_CURVE('',#4100,#4099,#496,.T.);
#5174=EDGE_CURVE('',#4098,#4100,#2642,.T.);
#5175=EDGE_CURVE('',#4101,#4097,#497,.T.);
#5176=EDGE_CURVE('',#4102,#4101,#2643,.T.);
#5177=EDGE_CURVE('',#4099,#4102,#498,.T.);
#5178=EDGE_CURVE('',#4103,#4104,#499,.T.);
#5179=EDGE_CURVE('',#4105,#4103,#2644,.T.);
#5180=EDGE_CURVE('',#4106,#4105,#500,.T.);
#5181=EDGE_CURVE('',#4104,#4106,#2645,.T.);
#5182=EDGE_CURVE('',#4107,#4103,#501,.T.);
#5183=EDGE_CURVE('',#4108,#4107,#2646,.T.);
#5184=EDGE_CURVE('',#4105,#4108,#502,.T.);
#5185=EDGE_CURVE('',#4109,#4110,#503,.T.);
#5186=EDGE_CURVE('',#4111,#4109,#2647,.T.);
#5187=EDGE_CURVE('',#4112,#4111,#504,.T.);
#5188=EDGE_CURVE('',#4110,#4112,#2648,.T.);
#5189=EDGE_CURVE('',#4113,#4109,#505,.T.);
#5190=EDGE_CURVE('',#4114,#4113,#2649,.T.);
#5191=EDGE_CURVE('',#4111,#4114,#506,.T.);
#5192=EDGE_CURVE('',#4115,#4116,#507,.T.);
#5193=EDGE_CURVE('',#4117,#4115,#2650,.T.);
#5194=EDGE_CURVE('',#4118,#4117,#508,.T.);
#5195=EDGE_CURVE('',#4116,#4118,#2651,.T.);
#5196=EDGE_CURVE('',#4119,#4115,#509,.T.);
#5197=EDGE_CURVE('',#4120,#4119,#2652,.T.);
#5198=EDGE_CURVE('',#4117,#4120,#510,.T.);
#5199=EDGE_CURVE('',#4121,#4122,#511,.T.);
#5200=EDGE_CURVE('',#4123,#4121,#2653,.T.);
#5201=EDGE_CURVE('',#4124,#4123,#512,.T.);
#5202=EDGE_CURVE('',#4122,#4124,#2654,.T.);
#5203=EDGE_CURVE('',#4125,#4121,#513,.T.);
#5204=EDGE_CURVE('',#4126,#4125,#2655,.T.);
#5205=EDGE_CURVE('',#4123,#4126,#514,.T.);
#5206=EDGE_CURVE('',#4127,#4128,#515,.T.);
#5207=EDGE_CURVE('',#4129,#4127,#2656,.T.);
#5208=EDGE_CURVE('',#4130,#4129,#516,.T.);
#5209=EDGE_CURVE('',#4128,#4130,#2657,.T.);
#5210=EDGE_CURVE('',#4131,#4127,#517,.T.);
#5211=EDGE_CURVE('',#4132,#4131,#2658,.T.);
#5212=EDGE_CURVE('',#4129,#4132,#518,.T.);
#5213=EDGE_CURVE('',#4133,#4134,#519,.T.);
#5214=EDGE_CURVE('',#4135,#4133,#2659,.T.);
#5215=EDGE_CURVE('',#4136,#4135,#520,.T.);
#5216=EDGE_CURVE('',#4134,#4136,#2660,.T.);
#5217=EDGE_CURVE('',#4137,#4133,#521,.T.);
#5218=EDGE_CURVE('',#4138,#4137,#2661,.T.);
#5219=EDGE_CURVE('',#4135,#4138,#522,.T.);
#5220=EDGE_CURVE('',#4139,#4140,#523,.T.);
#5221=EDGE_CURVE('',#4141,#4139,#2662,.T.);
#5222=EDGE_CURVE('',#4142,#4141,#524,.T.);
#5223=EDGE_CURVE('',#4140,#4142,#2663,.T.);
#5224=EDGE_CURVE('',#4143,#4139,#525,.T.);
#5225=EDGE_CURVE('',#4144,#4143,#2664,.T.);
#5226=EDGE_CURVE('',#4141,#4144,#526,.T.);
#5227=EDGE_CURVE('',#4145,#4146,#527,.T.);
#5228=EDGE_CURVE('',#4147,#4145,#2665,.T.);
#5229=EDGE_CURVE('',#4148,#4147,#528,.T.);
#5230=EDGE_CURVE('',#4146,#4148,#2666,.T.);
#5231=EDGE_CURVE('',#4149,#4145,#529,.T.);
#5232=EDGE_CURVE('',#4150,#4149,#2667,.T.);
#5233=EDGE_CURVE('',#4147,#4150,#530,.T.);
#5234=EDGE_CURVE('',#4151,#4152,#531,.T.);
#5235=EDGE_CURVE('',#4153,#4151,#2668,.T.);
#5236=EDGE_CURVE('',#4154,#4153,#532,.T.);
#5237=EDGE_CURVE('',#4152,#4154,#2669,.T.);
#5238=EDGE_CURVE('',#4155,#4151,#533,.T.);
#5239=EDGE_CURVE('',#4156,#4155,#2670,.T.);
#5240=EDGE_CURVE('',#4153,#4156,#534,.T.);
#5241=EDGE_CURVE('',#4157,#4158,#535,.T.);
#5242=EDGE_CURVE('',#4159,#4157,#2671,.T.);
#5243=EDGE_CURVE('',#4160,#4159,#536,.T.);
#5244=EDGE_CURVE('',#4158,#4160,#2672,.T.);
#5245=EDGE_CURVE('',#4161,#4157,#537,.T.);
#5246=EDGE_CURVE('',#4162,#4161,#2673,.T.);
#5247=EDGE_CURVE('',#4159,#4162,#538,.T.);
#5248=EDGE_CURVE('',#4163,#4164,#539,.T.);
#5249=EDGE_CURVE('',#4165,#4163,#2674,.T.);
#5250=EDGE_CURVE('',#4166,#4165,#540,.T.);
#5251=EDGE_CURVE('',#4164,#4166,#2675,.T.);
#5252=EDGE_CURVE('',#4167,#4163,#541,.T.);
#5253=EDGE_CURVE('',#4168,#4167,#2676,.T.);
#5254=EDGE_CURVE('',#4165,#4168,#542,.T.);
#5255=EDGE_CURVE('',#4169,#4170,#543,.T.);
#5256=EDGE_CURVE('',#4171,#4169,#2677,.T.);
#5257=EDGE_CURVE('',#4172,#4171,#544,.T.);
#5258=EDGE_CURVE('',#4170,#4172,#2678,.T.);
#5259=EDGE_CURVE('',#4173,#4169,#545,.T.);
#5260=EDGE_CURVE('',#4174,#4173,#2679,.T.);
#5261=EDGE_CURVE('',#4171,#4174,#546,.T.);
#5262=EDGE_CURVE('',#4175,#4176,#547,.T.);
#5263=EDGE_CURVE('',#4177,#4175,#2680,.T.);
#5264=EDGE_CURVE('',#4178,#4177,#548,.T.);
#5265=EDGE_CURVE('',#4176,#4178,#2681,.T.);
#5266=EDGE_CURVE('',#4179,#4175,#549,.T.);
#5267=EDGE_CURVE('',#4180,#4179,#2682,.T.);
#5268=EDGE_CURVE('',#4177,#4180,#550,.T.);
#5269=EDGE_CURVE('',#4181,#4182,#551,.T.);
#5270=EDGE_CURVE('',#4183,#4181,#2683,.T.);
#5271=EDGE_CURVE('',#4184,#4183,#552,.T.);
#5272=EDGE_CURVE('',#4182,#4184,#2684,.T.);
#5273=EDGE_CURVE('',#4185,#4181,#553,.T.);
#5274=EDGE_CURVE('',#4186,#4185,#2685,.T.);
#5275=EDGE_CURVE('',#4183,#4186,#554,.T.);
#5276=EDGE_CURVE('',#4187,#4188,#555,.T.);
#5277=EDGE_CURVE('',#4189,#4187,#2686,.T.);
#5278=EDGE_CURVE('',#4190,#4189,#556,.T.);
#5279=EDGE_CURVE('',#4188,#4190,#2687,.T.);
#5280=EDGE_CURVE('',#4191,#4187,#557,.T.);
#5281=EDGE_CURVE('',#4192,#4191,#2688,.T.);
#5282=EDGE_CURVE('',#4189,#4192,#558,.T.);
#5283=EDGE_CURVE('',#4032,#4185,#559,.T.);
#5284=EDGE_CURVE('',#4182,#4041,#560,.T.);
#5285=EDGE_CURVE('',#4038,#4179,#561,.T.);
#5286=EDGE_CURVE('',#4176,#4047,#562,.T.);
#5287=EDGE_CURVE('',#4044,#4173,#563,.T.);
#5288=EDGE_CURVE('',#4170,#4053,#564,.T.);
#5289=EDGE_CURVE('',#4050,#4167,#565,.T.);
#5290=EDGE_CURVE('',#4164,#4059,#566,.T.);
#5291=EDGE_CURVE('',#4056,#4161,#567,.T.);
#5292=EDGE_CURVE('',#4158,#4065,#568,.T.);
#5293=EDGE_CURVE('',#4062,#4155,#569,.T.);
#5294=EDGE_CURVE('',#4152,#4149,#570,.T.);
#5295=EDGE_CURVE('',#4146,#4077,#571,.T.);
#5296=EDGE_CURVE('',#4074,#4143,#572,.T.);
#5297=EDGE_CURVE('',#4140,#4083,#573,.T.);
#5298=EDGE_CURVE('',#4080,#4137,#574,.T.);
#5299=EDGE_CURVE('',#4134,#4089,#575,.T.);
#5300=EDGE_CURVE('',#4086,#4131,#576,.T.);
#5301=EDGE_CURVE('',#4128,#4095,#577,.T.);
#5302=EDGE_CURVE('',#4092,#4125,#578,.T.);
#5303=EDGE_CURVE('',#4122,#4101,#579,.T.);
#5304=EDGE_CURVE('',#4098,#4119,#580,.T.);
#5305=EDGE_CURVE('',#4116,#4107,#581,.T.);
#5306=EDGE_CURVE('',#4104,#4113,#582,.T.);
#5307=EDGE_CURVE('',#4110,#4071,#583,.T.);
#5308=EDGE_CURVE('',#4068,#4193,#584,.T.);
#5309=EDGE_CURVE('',#4193,#4194,#2689,.T.);
#5310=EDGE_CURVE('',#4195,#4194,#585,.T.);
#5311=EDGE_CURVE('',#4196,#4195,#2690,.T.);
#5312=EDGE_CURVE('',#4196,#4191,#586,.T.);
#5313=EDGE_CURVE('',#4188,#4035,#587,.T.);
#5314=EDGE_CURVE('',#4070,#4197,#588,.T.);
#5315=EDGE_CURVE('',#4197,#4193,#2691,.T.);
#5316=EDGE_CURVE('',#4198,#4196,#2692,.T.);
#5317=EDGE_CURVE('',#4199,#4198,#2693,.T.);
#5318=EDGE_CURVE('',#4200,#4199,#2694,.T.);
#5319=EDGE_CURVE('',#4201,#4200,#2695,.T.);
#5320=EDGE_CURVE('',#4201,#4192,#589,.T.);
#5321=EDGE_CURVE('',#4034,#4186,#590,.T.);
#5322=EDGE_CURVE('',#4040,#4180,#591,.T.);
#5323=EDGE_CURVE('',#4046,#4174,#592,.T.);
#5324=EDGE_CURVE('',#4052,#4168,#593,.T.);
#5325=EDGE_CURVE('',#4058,#4162,#594,.T.);
#5326=EDGE_CURVE('',#4064,#4156,#595,.T.);
#5327=EDGE_CURVE('',#4154,#4150,#596,.T.);
#5328=EDGE_CURVE('',#4076,#4144,#597,.T.);
#5329=EDGE_CURVE('',#4082,#4138,#598,.T.);
#5330=EDGE_CURVE('',#4088,#4132,#599,.T.);
#5331=EDGE_CURVE('',#4094,#4126,#600,.T.);
#5332=EDGE_CURVE('',#4100,#4120,#601,.T.);
#5333=EDGE_CURVE('',#4106,#4114,#602,.T.);
#5334=EDGE_CURVE('',#4118,#4108,#603,.T.);
#5335=EDGE_CURVE('',#4124,#4102,#604,.T.);
#5336=EDGE_CURVE('',#4130,#4096,#605,.T.);
#5337=EDGE_CURVE('',#4136,#4090,#606,.T.);
#5338=EDGE_CURVE('',#4142,#4084,#607,.T.);
#5339=EDGE_CURVE('',#4148,#4078,#608,.T.);
#5340=EDGE_CURVE('',#4112,#4072,#609,.T.);
#5341=EDGE_CURVE('',#4160,#4066,#610,.T.);
#5342=EDGE_CURVE('',#4166,#4060,#611,.T.);
#5343=EDGE_CURVE('',#4172,#4054,#612,.T.);
#5344=EDGE_CURVE('',#4178,#4048,#613,.T.);
#5345=EDGE_CURVE('',#4184,#4042,#614,.T.);
#5346=EDGE_CURVE('',#4202,#4197,#2696,.T.);
#5347=EDGE_CURVE('',#4194,#4202,#2697,.T.);
#5348=EDGE_CURVE('',#4198,#4203,#2698,.T.);
#5349=EDGE_CURVE('',#4195,#4203,#2699,.T.);
#5350=EDGE_CURVE('',#4204,#4202,#615,.T.);
#5351=EDGE_CURVE('',#4203,#4204,#2700,.T.);
#5352=EDGE_CURVE('',#4190,#4036,#616,.T.);
#5353=EDGE_CURVE('',#4204,#4201,#2701,.T.);
#5354=EDGE_CURVE('',#4203,#4205,#2702,.T.);
#5355=EDGE_CURVE('',#4206,#4204,#2703,.T.);
#5356=EDGE_CURVE('',#4205,#4206,#2704,.T.);
#5357=EDGE_CURVE('',#4207,#4208,#2705,.T.);
#5358=EDGE_CURVE('',#4205,#4207,#2706,.T.);
#5359=EDGE_CURVE('',#4208,#4206,#2707,.T.);
#5360=EDGE_CURVE('',#4199,#4209,#3675,.T.);
#5361=EDGE_CURVE('',#4209,#4210,#2708,.T.);
#5362=EDGE_CURVE('',#4200,#4210,#3676,.T.);
#5363=EDGE_CURVE('',#4211,#4208,#3677,.T.);
#5364=EDGE_CURVE('',#4211,#4212,#2709,.T.);
#5365=EDGE_CURVE('',#4212,#4207,#3678,.T.);
#5366=EDGE_CURVE('',#4210,#4213,#2710,.T.);
#5367=EDGE_CURVE('',#4213,#4214,#2711,.T.);
#5368=EDGE_CURVE('',#4214,#4215,#2712,.T.);
#5369=EDGE_CURVE('',#4215,#4216,#2713,.T.);
#5370=EDGE_CURVE('',#4216,#4217,#2714,.T.);
#5371=EDGE_CURVE('',#4217,#4211,#2715,.T.);
#5372=EDGE_CURVE('',#4209,#4218,#2716,.T.);
#5373=EDGE_CURVE('',#4218,#4213,#2717,.T.);
#5374=EDGE_CURVE('',#4219,#4217,#2718,.T.);
#5375=EDGE_CURVE('',#4219,#4212,#2719,.T.);
#5376=EDGE_CURVE('',#4220,#4219,#2720,.T.);
#5377=EDGE_CURVE('',#4220,#4216,#2721,.T.);
#5378=EDGE_CURVE('',#4221,#4220,#2722,.T.);
#5379=EDGE_CURVE('',#4221,#4215,#2723,.T.);
#5380=EDGE_CURVE('',#4222,#4221,#2724,.T.);
#5381=EDGE_CURVE('',#4222,#4214,#2725,.T.);
#5382=EDGE_CURVE('',#4218,#4222,#2726,.T.);
#6853=ORIENTED_EDGE('',*,*,#5085,.F.);
#6854=ORIENTED_EDGE('',*,*,#5086,.T.);
#6855=ORIENTED_EDGE('',*,*,#5087,.F.);
#6856=ORIENTED_EDGE('',*,*,#5086,.F.);
#6857=ORIENTED_EDGE('',*,*,#5088,.F.);
#6858=ORIENTED_EDGE('',*,*,#5089,.T.);
#6859=ORIENTED_EDGE('',*,*,#5090,.F.);
#6860=ORIENTED_EDGE('',*,*,#5089,.F.);
#6861=ORIENTED_EDGE('',*,*,#5091,.F.);
#6862=ORIENTED_EDGE('',*,*,#5092,.T.);
#6863=ORIENTED_EDGE('',*,*,#5093,.F.);
#6864=ORIENTED_EDGE('',*,*,#5092,.F.);
#6865=ORIENTED_EDGE('',*,*,#5094,.F.);
#6866=ORIENTED_EDGE('',*,*,#5095,.F.);
#6867=ORIENTED_EDGE('',*,*,#5096,.F.);
#6868=ORIENTED_EDGE('',*,*,#5097,.F.);
#6869=ORIENTED_EDGE('',*,*,#5098,.F.);
#6870=ORIENTED_EDGE('',*,*,#5099,.F.);
#6871=ORIENTED_EDGE('',*,*,#5100,.F.);
#6872=ORIENTED_EDGE('',*,*,#5095,.T.);
#6873=ORIENTED_EDGE('',*,*,#5101,.F.);
#6874=ORIENTED_EDGE('',*,*,#5102,.F.);
#6875=ORIENTED_EDGE('',*,*,#5103,.F.);
#6876=ORIENTED_EDGE('',*,*,#5104,.F.);
#6877=ORIENTED_EDGE('',*,*,#5105,.F.);
#6878=ORIENTED_EDGE('',*,*,#5106,.F.);
#6879=ORIENTED_EDGE('',*,*,#5107,.F.);
#6880=ORIENTED_EDGE('',*,*,#5102,.T.);
#6881=ORIENTED_EDGE('',*,*,#5108,.F.);
#6882=ORIENTED_EDGE('',*,*,#5109,.F.);
#6883=ORIENTED_EDGE('',*,*,#5110,.F.);
#6884=ORIENTED_EDGE('',*,*,#5111,.F.);
#6885=ORIENTED_EDGE('',*,*,#5112,.F.);
#6886=ORIENTED_EDGE('',*,*,#5113,.F.);
#6887=ORIENTED_EDGE('',*,*,#5114,.F.);
#6888=ORIENTED_EDGE('',*,*,#5109,.T.);
#6889=ORIENTED_EDGE('',*,*,#5115,.F.);
#6890=ORIENTED_EDGE('',*,*,#5116,.F.);
#6891=ORIENTED_EDGE('',*,*,#5117,.F.);
#6892=ORIENTED_EDGE('',*,*,#5118,.F.);
#6893=ORIENTED_EDGE('',*,*,#5119,.F.);
#6894=ORIENTED_EDGE('',*,*,#5120,.F.);
#6895=ORIENTED_EDGE('',*,*,#5121,.F.);
#6896=ORIENTED_EDGE('',*,*,#5116,.T.);
#6897=ORIENTED_EDGE('',*,*,#5122,.F.);
#6898=ORIENTED_EDGE('',*,*,#5123,.F.);
#6899=ORIENTED_EDGE('',*,*,#5124,.F.);
#6900=ORIENTED_EDGE('',*,*,#5125,.F.);
#6901=ORIENTED_EDGE('',*,*,#5126,.F.);
#6902=ORIENTED_EDGE('',*,*,#5127,.F.);
#6903=ORIENTED_EDGE('',*,*,#5128,.F.);
#6904=ORIENTED_EDGE('',*,*,#5123,.T.);
#6905=ORIENTED_EDGE('',*,*,#5129,.F.);
#6906=ORIENTED_EDGE('',*,*,#5130,.F.);
#6907=ORIENTED_EDGE('',*,*,#5131,.F.);
#6908=ORIENTED_EDGE('',*,*,#5132,.F.);
#6909=ORIENTED_EDGE('',*,*,#5133,.F.);
#6910=ORIENTED_EDGE('',*,*,#5134,.F.);
#6911=ORIENTED_EDGE('',*,*,#5135,.F.);
#6912=ORIENTED_EDGE('',*,*,#5130,.T.);
#6913=ORIENTED_EDGE('',*,*,#5136,.F.);
#6914=ORIENTED_EDGE('',*,*,#5137,.F.);
#6915=ORIENTED_EDGE('',*,*,#5138,.F.);
#6916=ORIENTED_EDGE('',*,*,#5139,.F.);
#6917=ORIENTED_EDGE('',*,*,#5140,.F.);
#6918=ORIENTED_EDGE('',*,*,#5141,.F.);
#6919=ORIENTED_EDGE('',*,*,#5142,.F.);
#6920=ORIENTED_EDGE('',*,*,#5137,.T.);
#6921=ORIENTED_EDGE('',*,*,#5143,.F.);
#6922=ORIENTED_EDGE('',*,*,#5144,.F.);
#6923=ORIENTED_EDGE('',*,*,#5145,.F.);
#6924=ORIENTED_EDGE('',*,*,#5146,.F.);
#6925=ORIENTED_EDGE('',*,*,#5147,.F.);
#6926=ORIENTED_EDGE('',*,*,#5148,.F.);
#6927=ORIENTED_EDGE('',*,*,#5149,.F.);
#6928=ORIENTED_EDGE('',*,*,#5144,.T.);
#6929=ORIENTED_EDGE('',*,*,#5150,.F.);
#6930=ORIENTED_EDGE('',*,*,#5151,.F.);
#6931=ORIENTED_EDGE('',*,*,#5152,.F.);
#6932=ORIENTED_EDGE('',*,*,#5153,.F.);
#6933=ORIENTED_EDGE('',*,*,#5154,.F.);
#6934=ORIENTED_EDGE('',*,*,#5155,.F.);
#6935=ORIENTED_EDGE('',*,*,#5156,.F.);
#6936=ORIENTED_EDGE('',*,*,#5151,.T.);
#6937=ORIENTED_EDGE('',*,*,#5157,.F.);
#6938=ORIENTED_EDGE('',*,*,#5158,.F.);
#6939=ORIENTED_EDGE('',*,*,#5159,.F.);
#6940=ORIENTED_EDGE('',*,*,#5160,.F.);
#6941=ORIENTED_EDGE('',*,*,#5161,.F.);
#6942=ORIENTED_EDGE('',*,*,#5162,.F.);
#6943=ORIENTED_EDGE('',*,*,#5163,.F.);
#6944=ORIENTED_EDGE('',*,*,#5158,.T.);
#6945=ORIENTED_EDGE('',*,*,#5164,.F.);
#6946=ORIENTED_EDGE('',*,*,#5165,.F.);
#6947=ORIENTED_EDGE('',*,*,#5166,.F.);
#6948=ORIENTED_EDGE('',*,*,#5167,.F.);
#6949=ORIENTED_EDGE('',*,*,#5168,.F.);
#6950=ORIENTED_EDGE('',*,*,#5169,.F.);
#6951=ORIENTED_EDGE('',*,*,#5170,.F.);
#6952=ORIENTED_EDGE('',*,*,#5165,.T.);
#6953=ORIENTED_EDGE('',*,*,#5171,.F.);
#6954=ORIENTED_EDGE('',*,*,#5172,.F.);
#6955=ORIENTED_EDGE('',*,*,#5173,.F.);
#6956=ORIENTED_EDGE('',*,*,#5174,.F.);
#6957=ORIENTED_EDGE('',*,*,#5175,.F.);
#6958=ORIENTED_EDGE('',*,*,#5176,.F.);
#6959=ORIENTED_EDGE('',*,*,#5177,.F.);
#6960=ORIENTED_EDGE('',*,*,#5172,.T.);
#6961=ORIENTED_EDGE('',*,*,#5178,.F.);
#6962=ORIENTED_EDGE('',*,*,#5179,.F.);
#6963=ORIENTED_EDGE('',*,*,#5180,.F.);
#6964=ORIENTED_EDGE('',*,*,#5181,.F.);
#6965=ORIENTED_EDGE('',*,*,#5182,.F.);
#6966=ORIENTED_EDGE('',*,*,#5183,.F.);
#6967=ORIENTED_EDGE('',*,*,#5184,.F.);
#6968=ORIENTED_EDGE('',*,*,#5179,.T.);
#6969=ORIENTED_EDGE('',*,*,#5185,.F.);
#6970=ORIENTED_EDGE('',*,*,#5186,.F.);
#6971=ORIENTED_EDGE('',*,*,#5187,.F.);
#6972=ORIENTED_EDGE('',*,*,#5188,.F.);
#6973=ORIENTED_EDGE('',*,*,#5189,.F.);
#6974=ORIENTED_EDGE('',*,*,#5190,.F.);
#6975=ORIENTED_EDGE('',*,*,#5191,.F.);
#6976=ORIENTED_EDGE('',*,*,#5186,.T.);
#6977=ORIENTED_EDGE('',*,*,#5192,.F.);
#6978=ORIENTED_EDGE('',*,*,#5193,.F.);
#6979=ORIENTED_EDGE('',*,*,#5194,.F.);
#6980=ORIENTED_EDGE('',*,*,#5195,.F.);
#6981=ORIENTED_EDGE('',*,*,#5196,.F.);
#6982=ORIENTED_EDGE('',*,*,#5197,.F.);
#6983=ORIENTED_EDGE('',*,*,#5198,.F.);
#6984=ORIENTED_EDGE('',*,*,#5193,.T.);
#6985=ORIENTED_EDGE('',*,*,#5199,.F.);
#6986=ORIENTED_EDGE('',*,*,#5200,.F.);
#6987=ORIENTED_EDGE('',*,*,#5201,.F.);
#6988=ORIENTED_EDGE('',*,*,#5202,.F.);
#6989=ORIENTED_EDGE('',*,*,#5203,.F.);
#6990=ORIENTED_EDGE('',*,*,#5204,.F.);
#6991=ORIENTED_EDGE('',*,*,#5205,.F.);
#6992=ORIENTED_EDGE('',*,*,#5200,.T.);
#6993=ORIENTED_EDGE('',*,*,#5206,.F.);
#6994=ORIENTED_EDGE('',*,*,#5207,.F.);
#6995=ORIENTED_EDGE('',*,*,#5208,.F.);
#6996=ORIENTED_EDGE('',*,*,#5209,.F.);
#6997=ORIENTED_EDGE('',*,*,#5210,.F.);
#6998=ORIENTED_EDGE('',*,*,#5211,.F.);
#6999=ORIENTED_EDGE('',*,*,#5212,.F.);
#7000=ORIENTED_EDGE('',*,*,#5207,.T.);
#7001=ORIENTED_EDGE('',*,*,#5213,.F.);
#7002=ORIENTED_EDGE('',*,*,#5214,.F.);
#7003=ORIENTED_EDGE('',*,*,#5215,.F.);
#7004=ORIENTED_EDGE('',*,*,#5216,.F.);
#7005=ORIENTED_EDGE('',*,*,#5217,.F.);
#7006=ORIENTED_EDGE('',*,*,#5218,.F.);
#7007=ORIENTED_EDGE('',*,*,#5219,.F.);
#7008=ORIENTED_EDGE('',*,*,#5214,.T.);
#7009=ORIENTED_EDGE('',*,*,#5220,.F.);
#7010=ORIENTED_EDGE('',*,*,#5221,.F.);
#7011=ORIENTED_EDGE('',*,*,#5222,.F.);
#7012=ORIENTED_EDGE('',*,*,#5223,.F.);
#7013=ORIENTED_EDGE('',*,*,#5224,.F.);
#7014=ORIENTED_EDGE('',*,*,#5225,.F.);
#7015=ORIENTED_EDGE('',*,*,#5226,.F.);
#7016=ORIENTED_EDGE('',*,*,#5221,.T.);
#7017=ORIENTED_EDGE('',*,*,#5227,.F.);
#7018=ORIENTED_EDGE('',*,*,#5228,.F.);
#7019=ORIENTED_EDGE('',*,*,#5229,.F.);
#7020=ORIENTED_EDGE('',*,*,#5230,.F.);
#7021=ORIENTED_EDGE('',*,*,#5231,.F.);
#7022=ORIENTED_EDGE('',*,*,#5232,.F.);
#7023=ORIENTED_EDGE('',*,*,#5233,.F.);
#7024=ORIENTED_EDGE('',*,*,#5228,.T.);
#7025=ORIENTED_EDGE('',*,*,#5234,.F.);
#7026=ORIENTED_EDGE('',*,*,#5235,.F.);
#7027=ORIENTED_EDGE('',*,*,#5236,.F.);
#7028=ORIENTED_EDGE('',*,*,#5237,.F.);
#7029=ORIENTED_EDGE('',*,*,#5238,.F.);
#7030=ORIENTED_EDGE('',*,*,#5239,.F.);
#7031=ORIENTED_EDGE('',*,*,#5240,.F.);
#7032=ORIENTED_EDGE('',*,*,#5235,.T.);
#7033=ORIENTED_EDGE('',*,*,#5241,.F.);
#7034=ORIENTED_EDGE('',*,*,#5242,.F.);
#7035=ORIENTED_EDGE('',*,*,#5243,.F.);
#7036=ORIENTED_EDGE('',*,*,#5244,.F.);
#7037=ORIENTED_EDGE('',*,*,#5245,.F.);
#7038=ORIENTED_EDGE('',*,*,#5246,.F.);
#7039=ORIENTED_EDGE('',*,*,#5247,.F.);
#7040=ORIENTED_EDGE('',*,*,#5242,.T.);
#7041=ORIENTED_EDGE('',*,*,#5248,.F.);
#7042=ORIENTED_EDGE('',*,*,#5249,.F.);
#7043=ORIENTED_EDGE('',*,*,#5250,.F.);
#7044=ORIENTED_EDGE('',*,*,#5251,.F.);
#7045=ORIENTED_EDGE('',*,*,#5252,.F.);
#7046=ORIENTED_EDGE('',*,*,#5253,.F.);
#7047=ORIENTED_EDGE('',*,*,#5254,.F.);
#7048=ORIENTED_EDGE('',*,*,#5249,.T.);
#7049=ORIENTED_EDGE('',*,*,#5255,.F.);
#7050=ORIENTED_EDGE('',*,*,#5256,.F.);
#7051=ORIENTED_EDGE('',*,*,#5257,.F.);
#7052=ORIENTED_EDGE('',*,*,#5258,.F.);
#7053=ORIENTED_EDGE('',*,*,#5259,.F.);
#7054=ORIENTED_EDGE('',*,*,#5260,.F.);
#7055=ORIENTED_EDGE('',*,*,#5261,.F.);
#7056=ORIENTED_EDGE('',*,*,#5256,.T.);
#7057=ORIENTED_EDGE('',*,*,#5262,.F.);
#7058=ORIENTED_EDGE('',*,*,#5263,.F.);
#7059=ORIENTED_EDGE('',*,*,#5264,.F.);
#7060=ORIENTED_EDGE('',*,*,#5265,.F.);
#7061=ORIENTED_EDGE('',*,*,#5266,.F.);
#7062=ORIENTED_EDGE('',*,*,#5267,.F.);
#7063=ORIENTED_EDGE('',*,*,#5268,.F.);
#7064=ORIENTED_EDGE('',*,*,#5263,.T.);
#7065=ORIENTED_EDGE('',*,*,#5269,.F.);
#7066=ORIENTED_EDGE('',*,*,#5270,.F.);
#7067=ORIENTED_EDGE('',*,*,#5271,.F.);
#7068=ORIENTED_EDGE('',*,*,#5272,.F.);
#7069=ORIENTED_EDGE('',*,*,#5273,.F.);
#7070=ORIENTED_EDGE('',*,*,#5274,.F.);
#7071=ORIENTED_EDGE('',*,*,#5275,.F.);
#7072=ORIENTED_EDGE('',*,*,#5270,.T.);
#7073=ORIENTED_EDGE('',*,*,#5276,.F.);
#7074=ORIENTED_EDGE('',*,*,#5277,.F.);
#7075=ORIENTED_EDGE('',*,*,#5278,.F.);
#7076=ORIENTED_EDGE('',*,*,#5279,.F.);
#7077=ORIENTED_EDGE('',*,*,#5280,.F.);
#7078=ORIENTED_EDGE('',*,*,#5281,.F.);
#7079=ORIENTED_EDGE('',*,*,#5282,.F.);
#7080=ORIENTED_EDGE('',*,*,#5277,.T.);
#7081=ORIENTED_EDGE('',*,*,#5098,.T.);
#7082=ORIENTED_EDGE('',*,*,#5094,.T.);
#7083=ORIENTED_EDGE('',*,*,#5283,.T.);
#7084=ORIENTED_EDGE('',*,*,#5273,.T.);
#7085=ORIENTED_EDGE('',*,*,#5269,.T.);
#7086=ORIENTED_EDGE('',*,*,#5284,.T.);
#7087=ORIENTED_EDGE('',*,*,#5105,.T.);
#7088=ORIENTED_EDGE('',*,*,#5101,.T.);
#7089=ORIENTED_EDGE('',*,*,#5285,.T.);
#7090=ORIENTED_EDGE('',*,*,#5266,.T.);
#7091=ORIENTED_EDGE('',*,*,#5262,.T.);
#7092=ORIENTED_EDGE('',*,*,#5286,.T.);
#7093=ORIENTED_EDGE('',*,*,#5112,.T.);
#7094=ORIENTED_EDGE('',*,*,#5108,.T.);
#7095=ORIENTED_EDGE('',*,*,#5287,.T.);
#7096=ORIENTED_EDGE('',*,*,#5259,.T.);
#7097=ORIENTED_EDGE('',*,*,#5255,.T.);
#7098=ORIENTED_EDGE('',*,*,#5288,.T.);
#7099=ORIENTED_EDGE('',*,*,#5119,.T.);
#7100=ORIENTED_EDGE('',*,*,#5115,.T.);
#7101=ORIENTED_EDGE('',*,*,#5289,.T.);
#7102=ORIENTED_EDGE('',*,*,#5252,.T.);
#7103=ORIENTED_EDGE('',*,*,#5248,.T.);
#7104=ORIENTED_EDGE('',*,*,#5290,.T.);
#7105=ORIENTED_EDGE('',*,*,#5126,.T.);
#7106=ORIENTED_EDGE('',*,*,#5122,.T.);
#7107=ORIENTED_EDGE('',*,*,#5291,.T.);
#7108=ORIENTED_EDGE('',*,*,#5245,.T.);
#7109=ORIENTED_EDGE('',*,*,#5241,.T.);
#7110=ORIENTED_EDGE('',*,*,#5292,.T.);
#7111=ORIENTED_EDGE('',*,*,#5133,.T.);
#7112=ORIENTED_EDGE('',*,*,#5129,.T.);
#7113=ORIENTED_EDGE('',*,*,#5293,.T.);
#7114=ORIENTED_EDGE('',*,*,#5238,.T.);
#7115=ORIENTED_EDGE('',*,*,#5234,.T.);
#7116=ORIENTED_EDGE('',*,*,#5294,.T.);
#7117=ORIENTED_EDGE('',*,*,#5231,.T.);
#7118=ORIENTED_EDGE('',*,*,#5227,.T.);
#7119=ORIENTED_EDGE('',*,*,#5295,.T.);
#7120=ORIENTED_EDGE('',*,*,#5147,.T.);
#7121=ORIENTED_EDGE('',*,*,#5143,.T.);
#7122=ORIENTED_EDGE('',*,*,#5296,.T.);
#7123=ORIENTED_EDGE('',*,*,#5224,.T.);
#7124=ORIENTED_EDGE('',*,*,#5220,.T.);
#7125=ORIENTED_EDGE('',*,*,#5297,.T.);
#7126=ORIENTED_EDGE('',*,*,#5154,.T.);
#7127=ORIENTED_EDGE('',*,*,#5150,.T.);
#7128=ORIENTED_EDGE('',*,*,#5298,.T.);
#7129=ORIENTED_EDGE('',*,*,#5217,.T.);
#7130=ORIENTED_EDGE('',*,*,#5213,.T.);
#7131=ORIENTED_EDGE('',*,*,#5299,.T.);
#7132=ORIENTED_EDGE('',*,*,#5161,.T.);
#7133=ORIENTED_EDGE('',*,*,#5157,.T.);
#7134=ORIENTED_EDGE('',*,*,#5300,.T.);
#7135=ORIENTED_EDGE('',*,*,#5210,.T.);
#7136=ORIENTED_EDGE('',*,*,#5206,.T.);
#7137=ORIENTED_EDGE('',*,*,#5301,.T.);
#7138=ORIENTED_EDGE('',*,*,#5168,.T.);
#7139=ORIENTED_EDGE('',*,*,#5164,.T.);
#7140=ORIENTED_EDGE('',*,*,#5302,.T.);
#7141=ORIENTED_EDGE('',*,*,#5203,.T.);
#7142=ORIENTED_EDGE('',*,*,#5199,.T.);
#7143=ORIENTED_EDGE('',*,*,#5303,.T.);
#7144=ORIENTED_EDGE('',*,*,#5175,.T.);
#7145=ORIENTED_EDGE('',*,*,#5171,.T.);
#7146=ORIENTED_EDGE('',*,*,#5304,.T.);
#7147=ORIENTED_EDGE('',*,*,#5196,.T.);
#7148=ORIENTED_EDGE('',*,*,#5192,.T.);
#7149=ORIENTED_EDGE('',*,*,#5305,.T.);
#7150=ORIENTED_EDGE('',*,*,#5182,.T.);
#7151=ORIENTED_EDGE('',*,*,#5178,.T.);
#7152=ORIENTED_EDGE('',*,*,#5306,.T.);
#7153=ORIENTED_EDGE('',*,*,#5189,.T.);
#7154=ORIENTED_EDGE('',*,*,#5185,.T.);
#7155=ORIENTED_EDGE('',*,*,#5307,.T.);
#7156=ORIENTED_EDGE('',*,*,#5140,.T.);
#7157=ORIENTED_EDGE('',*,*,#5136,.T.);
#7158=ORIENTED_EDGE('',*,*,#5308,.T.);
#7159=ORIENTED_EDGE('',*,*,#5309,.T.);
#7160=ORIENTED_EDGE('',*,*,#5310,.F.);
#7161=ORIENTED_EDGE('',*,*,#5311,.F.);
#7162=ORIENTED_EDGE('',*,*,#5312,.T.);
#7163=ORIENTED_EDGE('',*,*,#5280,.T.);
#7164=ORIENTED_EDGE('',*,*,#5276,.T.);
#7165=ORIENTED_EDGE('',*,*,#5313,.T.);
#7166=ORIENTED_EDGE('',*,*,#5139,.T.);
#7167=ORIENTED_EDGE('',*,*,#5314,.T.);
#7168=ORIENTED_EDGE('',*,*,#5315,.T.);
#7169=ORIENTED_EDGE('',*,*,#5308,.F.);
#7170=ORIENTED_EDGE('',*,*,#5281,.T.);
#7171=ORIENTED_EDGE('',*,*,#5312,.F.);
#7172=ORIENTED_EDGE('',*,*,#5316,.F.);
#7173=ORIENTED_EDGE('',*,*,#5317,.F.);
#7174=ORIENTED_EDGE('',*,*,#5318,.F.);
#7175=ORIENTED_EDGE('',*,*,#5319,.F.);
#7176=ORIENTED_EDGE('',*,*,#5320,.T.);
#7177=ORIENTED_EDGE('',*,*,#5097,.T.);
#7178=ORIENTED_EDGE('',*,*,#5321,.T.);
#7179=ORIENTED_EDGE('',*,*,#5274,.T.);
#7180=ORIENTED_EDGE('',*,*,#5283,.F.);
#7181=ORIENTED_EDGE('',*,*,#5104,.T.);
#7182=ORIENTED_EDGE('',*,*,#5322,.T.);
#7183=ORIENTED_EDGE('',*,*,#5267,.T.);
#7184=ORIENTED_EDGE('',*,*,#5285,.F.);
#7185=ORIENTED_EDGE('',*,*,#5111,.T.);
#7186=ORIENTED_EDGE('',*,*,#5323,.T.);
#7187=ORIENTED_EDGE('',*,*,#5260,.T.);
#7188=ORIENTED_EDGE('',*,*,#5287,.F.);
#7189=ORIENTED_EDGE('',*,*,#5118,.T.);
#7190=ORIENTED_EDGE('',*,*,#5324,.T.);
#7191=ORIENTED_EDGE('',*,*,#5253,.T.);
#7192=ORIENTED_EDGE('',*,*,#5289,.F.);
#7193=ORIENTED_EDGE('',*,*,#5125,.T.);
#7194=ORIENTED_EDGE('',*,*,#5325,.T.);
#7195=ORIENTED_EDGE('',*,*,#5246,.T.);
#7196=ORIENTED_EDGE('',*,*,#5291,.F.);
#7197=ORIENTED_EDGE('',*,*,#5132,.T.);
#7198=ORIENTED_EDGE('',*,*,#5326,.T.);
#7199=ORIENTED_EDGE('',*,*,#5239,.T.);
#7200=ORIENTED_EDGE('',*,*,#5293,.F.);
#7201=ORIENTED_EDGE('',*,*,#5232,.T.);
#7202=ORIENTED_EDGE('',*,*,#5294,.F.);
#7203=ORIENTED_EDGE('',*,*,#5237,.T.);
#7204=ORIENTED_EDGE('',*,*,#5327,.T.);
#7205=ORIENTED_EDGE('',*,*,#5146,.T.);
#7206=ORIENTED_EDGE('',*,*,#5328,.T.);
#7207=ORIENTED_EDGE('',*,*,#5225,.T.);
#7208=ORIENTED_EDGE('',*,*,#5296,.F.);
#7209=ORIENTED_EDGE('',*,*,#5153,.T.);
#7210=ORIENTED_EDGE('',*,*,#5329,.T.);
#7211=ORIENTED_EDGE('',*,*,#5218,.T.);
#7212=ORIENTED_EDGE('',*,*,#5298,.F.);
#7213=ORIENTED_EDGE('',*,*,#5160,.T.);
#7214=ORIENTED_EDGE('',*,*,#5330,.T.);
#7215=ORIENTED_EDGE('',*,*,#5211,.T.);
#7216=ORIENTED_EDGE('',*,*,#5300,.F.);
#7217=ORIENTED_EDGE('',*,*,#5167,.T.);
#7218=ORIENTED_EDGE('',*,*,#5331,.T.);
#7219=ORIENTED_EDGE('',*,*,#5204,.T.);
#7220=ORIENTED_EDGE('',*,*,#5302,.F.);
#7221=ORIENTED_EDGE('',*,*,#5174,.T.);
#7222=ORIENTED_EDGE('',*,*,#5332,.T.);
#7223=ORIENTED_EDGE('',*,*,#5197,.T.);
#7224=ORIENTED_EDGE('',*,*,#5304,.F.);
#7225=ORIENTED_EDGE('',*,*,#5181,.T.);
#7226=ORIENTED_EDGE('',*,*,#5333,.T.);
#7227=ORIENTED_EDGE('',*,*,#5190,.T.);
#7228=ORIENTED_EDGE('',*,*,#5306,.F.);
#7229=ORIENTED_EDGE('',*,*,#5183,.T.);
#7230=ORIENTED_EDGE('',*,*,#5305,.F.);
#7231=ORIENTED_EDGE('',*,*,#5195,.T.);
#7232=ORIENTED_EDGE('',*,*,#5334,.T.);
#7233=ORIENTED_EDGE('',*,*,#5176,.T.);
#7234=ORIENTED_EDGE('',*,*,#5303,.F.);
#7235=ORIENTED_EDGE('',*,*,#5202,.T.);
#7236=ORIENTED_EDGE('',*,*,#5335,.T.);
#7237=ORIENTED_EDGE('',*,*,#5169,.T.);
#7238=ORIENTED_EDGE('',*,*,#5301,.F.);
#7239=ORIENTED_EDGE('',*,*,#5209,.T.);
#7240=ORIENTED_EDGE('',*,*,#5336,.T.);
#7241=ORIENTED_EDGE('',*,*,#5162,.T.);
#7242=ORIENTED_EDGE('',*,*,#5299,.F.);
#7243=ORIENTED_EDGE('',*,*,#5216,.T.);
#7244=ORIENTED_EDGE('',*,*,#5337,.T.);
#7245=ORIENTED_EDGE('',*,*,#5155,.T.);
#7246=ORIENTED_EDGE('',*,*,#5297,.F.);
#7247=ORIENTED_EDGE('',*,*,#5223,.T.);
#7248=ORIENTED_EDGE('',*,*,#5338,.T.);
#7249=ORIENTED_EDGE('',*,*,#5148,.T.);
#7250=ORIENTED_EDGE('',*,*,#5295,.F.);
#7251=ORIENTED_EDGE('',*,*,#5230,.T.);
#7252=ORIENTED_EDGE('',*,*,#5339,.T.);
#7253=ORIENTED_EDGE('',*,*,#5141,.T.);
#7254=ORIENTED_EDGE('',*,*,#5307,.F.);
#7255=ORIENTED_EDGE('',*,*,#5188,.T.);
#7256=ORIENTED_EDGE('',*,*,#5340,.T.);
#7257=ORIENTED_EDGE('',*,*,#5134,.T.);
#7258=ORIENTED_EDGE('',*,*,#5292,.F.);
#7259=ORIENTED_EDGE('',*,*,#5244,.T.);
#7260=ORIENTED_EDGE('',*,*,#5341,.T.);
#7261=ORIENTED_EDGE('',*,*,#5127,.T.);
#7262=ORIENTED_EDGE('',*,*,#5290,.F.);
#7263=ORIENTED_EDGE('',*,*,#5251,.T.);
#7264=ORIENTED_EDGE('',*,*,#5342,.T.);
#7265=ORIENTED_EDGE('',*,*,#5120,.T.);
#7266=ORIENTED_EDGE('',*,*,#5288,.F.);
#7267=ORIENTED_EDGE('',*,*,#5258,.T.);
#7268=ORIENTED_EDGE('',*,*,#5343,.T.);
#7269=ORIENTED_EDGE('',*,*,#5113,.T.);
#7270=ORIENTED_EDGE('',*,*,#5286,.F.);
#7271=ORIENTED_EDGE('',*,*,#5265,.T.);
#7272=ORIENTED_EDGE('',*,*,#5344,.T.);
#7273=ORIENTED_EDGE('',*,*,#5106,.T.);
#7274=ORIENTED_EDGE('',*,*,#5284,.F.);
#7275=ORIENTED_EDGE('',*,*,#5272,.T.);
#7276=ORIENTED_EDGE('',*,*,#5345,.T.);
#7277=ORIENTED_EDGE('',*,*,#5315,.F.);
#7278=ORIENTED_EDGE('',*,*,#5346,.F.);
#7279=ORIENTED_EDGE('',*,*,#5347,.F.);
#7280=ORIENTED_EDGE('',*,*,#5309,.F.);
#7281=ORIENTED_EDGE('',*,*,#5348,.F.);
#7282=ORIENTED_EDGE('',*,*,#5316,.T.);
#7283=ORIENTED_EDGE('',*,*,#5311,.T.);
#7284=ORIENTED_EDGE('',*,*,#5349,.T.);
#7285=ORIENTED_EDGE('',*,*,#5349,.F.);
#7286=ORIENTED_EDGE('',*,*,#5310,.T.);
#7287=ORIENTED_EDGE('',*,*,#5347,.T.);
#7288=ORIENTED_EDGE('',*,*,#5350,.F.);
#7289=ORIENTED_EDGE('',*,*,#5351,.F.);
#7290=ORIENTED_EDGE('',*,*,#5100,.T.);
#7291=ORIENTED_EDGE('',*,*,#5352,.F.);
#7292=ORIENTED_EDGE('',*,*,#5278,.T.);
#7293=ORIENTED_EDGE('',*,*,#5282,.T.);
#7294=ORIENTED_EDGE('',*,*,#5320,.F.);
#7295=ORIENTED_EDGE('',*,*,#5353,.F.);
#7296=ORIENTED_EDGE('',*,*,#5350,.T.);
#7297=ORIENTED_EDGE('',*,*,#5346,.T.);
#7298=ORIENTED_EDGE('',*,*,#5314,.F.);
#7299=ORIENTED_EDGE('',*,*,#5138,.T.);
#7300=ORIENTED_EDGE('',*,*,#5142,.T.);
#7301=ORIENTED_EDGE('',*,*,#5340,.F.);
#7302=ORIENTED_EDGE('',*,*,#5187,.T.);
#7303=ORIENTED_EDGE('',*,*,#5191,.T.);
#7304=ORIENTED_EDGE('',*,*,#5333,.F.);
#7305=ORIENTED_EDGE('',*,*,#5180,.T.);
#7306=ORIENTED_EDGE('',*,*,#5184,.T.);
#7307=ORIENTED_EDGE('',*,*,#5334,.F.);
#7308=ORIENTED_EDGE('',*,*,#5194,.T.);
#7309=ORIENTED_EDGE('',*,*,#5198,.T.);
#7310=ORIENTED_EDGE('',*,*,#5332,.F.);
#7311=ORIENTED_EDGE('',*,*,#5173,.T.);
#7312=ORIENTED_EDGE('',*,*,#5177,.T.);
#7313=ORIENTED_EDGE('',*,*,#5335,.F.);
#7314=ORIENTED_EDGE('',*,*,#5201,.T.);
#7315=ORIENTED_EDGE('',*,*,#5205,.T.);
#7316=ORIENTED_EDGE('',*,*,#5331,.F.);
#7317=ORIENTED_EDGE('',*,*,#5166,.T.);
#7318=ORIENTED_EDGE('',*,*,#5170,.T.);
#7319=ORIENTED_EDGE('',*,*,#5336,.F.);
#7320=ORIENTED_EDGE('',*,*,#5208,.T.);
#7321=ORIENTED_EDGE('',*,*,#5212,.T.);
#7322=ORIENTED_EDGE('',*,*,#5330,.F.);
#7323=ORIENTED_EDGE('',*,*,#5159,.T.);
#7324=ORIENTED_EDGE('',*,*,#5163,.T.);
#7325=ORIENTED_EDGE('',*,*,#5337,.F.);
#7326=ORIENTED_EDGE('',*,*,#5215,.T.);
#7327=ORIENTED_EDGE('',*,*,#5219,.T.);
#7328=ORIENTED_EDGE('',*,*,#5329,.F.);
#7329=ORIENTED_EDGE('',*,*,#5152,.T.);
#7330=ORIENTED_EDGE('',*,*,#5156,.T.);
#7331=ORIENTED_EDGE('',*,*,#5338,.F.);
#7332=ORIENTED_EDGE('',*,*,#5222,.T.);
#7333=ORIENTED_EDGE('',*,*,#5226,.T.);
#7334=ORIENTED_EDGE('',*,*,#5328,.F.);
#7335=ORIENTED_EDGE('',*,*,#5145,.T.);
#7336=ORIENTED_EDGE('',*,*,#5149,.T.);
#7337=ORIENTED_EDGE('',*,*,#5339,.F.);
#7338=ORIENTED_EDGE('',*,*,#5229,.T.);
#7339=ORIENTED_EDGE('',*,*,#5233,.T.);
#7340=ORIENTED_EDGE('',*,*,#5327,.F.);
#7341=ORIENTED_EDGE('',*,*,#5236,.T.);
#7342=ORIENTED_EDGE('',*,*,#5240,.T.);
#7343=ORIENTED_EDGE('',*,*,#5326,.F.);
#7344=ORIENTED_EDGE('',*,*,#5131,.T.);
#7345=ORIENTED_EDGE('',*,*,#5135,.T.);
#7346=ORIENTED_EDGE('',*,*,#5341,.F.);
#7347=ORIENTED_EDGE('',*,*,#5243,.T.);
#7348=ORIENTED_EDGE('',*,*,#5247,.T.);
#7349=ORIENTED_EDGE('',*,*,#5325,.F.);
#7350=ORIENTED_EDGE('',*,*,#5124,.T.);
#7351=ORIENTED_EDGE('',*,*,#5128,.T.);
#7352=ORIENTED_EDGE('',*,*,#5342,.F.);
#7353=ORIENTED_EDGE('',*,*,#5250,.T.);
#7354=ORIENTED_EDGE('',*,*,#5254,.T.);
#7355=ORIENTED_EDGE('',*,*,#5324,.F.);
#7356=ORIENTED_EDGE('',*,*,#5117,.T.);
#7357=ORIENTED_EDGE('',*,*,#5121,.T.);
#7358=ORIENTED_EDGE('',*,*,#5343,.F.);
#7359=ORIENTED_EDGE('',*,*,#5257,.T.);
#7360=ORIENTED_EDGE('',*,*,#5261,.T.);
#7361=ORIENTED_EDGE('',*,*,#5323,.F.);
#7362=ORIENTED_EDGE('',*,*,#5110,.T.);
#7363=ORIENTED_EDGE('',*,*,#5114,.T.);
#7364=ORIENTED_EDGE('',*,*,#5344,.F.);
#7365=ORIENTED_EDGE('',*,*,#5264,.T.);
#7366=ORIENTED_EDGE('',*,*,#5268,.T.);
#7367=ORIENTED_EDGE('',*,*,#5322,.F.);
#7368=ORIENTED_EDGE('',*,*,#5103,.T.);
#7369=ORIENTED_EDGE('',*,*,#5107,.T.);
#7370=ORIENTED_EDGE('',*,*,#5345,.F.);
#7371=ORIENTED_EDGE('',*,*,#5271,.T.);
#7372=ORIENTED_EDGE('',*,*,#5275,.T.);
#7373=ORIENTED_EDGE('',*,*,#5321,.F.);
#7374=ORIENTED_EDGE('',*,*,#5096,.T.);
#7375=ORIENTED_EDGE('',*,*,#5099,.T.);
#7376=ORIENTED_EDGE('',*,*,#5313,.F.);
#7377=ORIENTED_EDGE('',*,*,#5279,.T.);
#7378=ORIENTED_EDGE('',*,*,#5352,.T.);
#7379=ORIENTED_EDGE('',*,*,#5354,.F.);
#7380=ORIENTED_EDGE('',*,*,#5351,.T.);
#7381=ORIENTED_EDGE('',*,*,#5355,.F.);
#7382=ORIENTED_EDGE('',*,*,#5356,.F.);
#7383=ORIENTED_EDGE('',*,*,#5357,.F.);
#7384=ORIENTED_EDGE('',*,*,#5358,.F.);
#7385=ORIENTED_EDGE('',*,*,#5356,.T.);
#7386=ORIENTED_EDGE('',*,*,#5359,.F.);
#7387=ORIENTED_EDGE('',*,*,#5318,.T.);
#7388=ORIENTED_EDGE('',*,*,#5360,.T.);
#7389=ORIENTED_EDGE('',*,*,#5361,.T.);
#7390=ORIENTED_EDGE('',*,*,#5362,.F.);
#7391=ORIENTED_EDGE('',*,*,#5357,.T.);
#7392=ORIENTED_EDGE('',*,*,#5363,.F.);
#7393=ORIENTED_EDGE('',*,*,#5364,.T.);
#7394=ORIENTED_EDGE('',*,*,#5365,.T.);
#7395=ORIENTED_EDGE('',*,*,#5362,.T.);
#7396=ORIENTED_EDGE('',*,*,#5366,.T.);
#7397=ORIENTED_EDGE('',*,*,#5367,.T.);
#7398=ORIENTED_EDGE('',*,*,#5368,.T.);
#7399=ORIENTED_EDGE('',*,*,#5369,.T.);
#7400=ORIENTED_EDGE('',*,*,#5370,.T.);
#7401=ORIENTED_EDGE('',*,*,#5371,.T.);
#7402=ORIENTED_EDGE('',*,*,#5363,.T.);
#7403=ORIENTED_EDGE('',*,*,#5359,.T.);
#7404=ORIENTED_EDGE('',*,*,#5355,.T.);
#7405=ORIENTED_EDGE('',*,*,#5353,.T.);
#7406=ORIENTED_EDGE('',*,*,#5319,.T.);
#7407=ORIENTED_EDGE('',*,*,#5085,.T.);
#7408=ORIENTED_EDGE('',*,*,#5088,.T.);
#7409=ORIENTED_EDGE('',*,*,#5091,.T.);
#7410=ORIENTED_EDGE('',*,*,#5361,.F.);
#7411=ORIENTED_EDGE('',*,*,#5372,.T.);
#7412=ORIENTED_EDGE('',*,*,#5373,.T.);
#7413=ORIENTED_EDGE('',*,*,#5366,.F.);
#7414=ORIENTED_EDGE('',*,*,#5364,.F.);
#7415=ORIENTED_EDGE('',*,*,#5371,.F.);
#7416=ORIENTED_EDGE('',*,*,#5374,.F.);
#7417=ORIENTED_EDGE('',*,*,#5375,.T.);
#7418=ORIENTED_EDGE('',*,*,#5376,.T.);
#7419=ORIENTED_EDGE('',*,*,#5374,.T.);
#7420=ORIENTED_EDGE('',*,*,#5370,.F.);
#7421=ORIENTED_EDGE('',*,*,#5377,.F.);
#7422=ORIENTED_EDGE('',*,*,#5378,.T.);
#7423=ORIENTED_EDGE('',*,*,#5377,.T.);
#7424=ORIENTED_EDGE('',*,*,#5369,.F.);
#7425=ORIENTED_EDGE('',*,*,#5379,.F.);
#7426=ORIENTED_EDGE('',*,*,#5380,.T.);
#7427=ORIENTED_EDGE('',*,*,#5379,.T.);
#7428=ORIENTED_EDGE('',*,*,#5368,.F.);
#7429=ORIENTED_EDGE('',*,*,#5381,.F.);
#7430=ORIENTED_EDGE('',*,*,#5382,.T.);
#7431=ORIENTED_EDGE('',*,*,#5381,.T.);
#7432=ORIENTED_EDGE('',*,*,#5367,.F.);
#7433=ORIENTED_EDGE('',*,*,#5373,.F.);
#7434=ORIENTED_EDGE('',*,*,#5365,.F.);
#7435=ORIENTED_EDGE('',*,*,#5375,.F.);
#7436=ORIENTED_EDGE('',*,*,#5376,.F.);
#7437=ORIENTED_EDGE('',*,*,#5378,.F.);
#7438=ORIENTED_EDGE('',*,*,#5380,.F.);
#7439=ORIENTED_EDGE('',*,*,#5382,.F.);
#7440=ORIENTED_EDGE('',*,*,#5372,.F.);
#7441=ORIENTED_EDGE('',*,*,#5360,.F.);
#7442=ORIENTED_EDGE('',*,*,#5317,.T.);
#7443=ORIENTED_EDGE('',*,*,#5348,.T.);
#7444=ORIENTED_EDGE('',*,*,#5354,.T.);
#7445=ORIENTED_EDGE('',*,*,#5358,.T.);
#7446=ORIENTED_EDGE('',*,*,#5087,.T.);
#7447=ORIENTED_EDGE('',*,*,#5090,.T.);
#7448=ORIENTED_EDGE('',*,*,#5093,.T.);
#9202=CYLINDRICAL_SURFACE('',#10122,0.17);
#9203=CYLINDRICAL_SURFACE('',#10125,0.17);
#9204=CYLINDRICAL_SURFACE('',#10128,0.41);
#9205=CYLINDRICAL_SURFACE('',#10217,1.4);
#9206=CYLINDRICAL_SURFACE('',#10220,1.4);
#9438=ADVANCED_FACE('',(#1412),#9202,.F.);
#9439=ADVANCED_FACE('',(#1413),#9203,.F.);
#9440=ADVANCED_FACE('',(#1414),#9204,.F.);
#9441=ADVANCED_FACE('',(#1415),#1093,.F.);
#9442=ADVANCED_FACE('',(#1416),#1094,.F.);
#9443=ADVANCED_FACE('',(#1417),#1095,.F.);
#9444=ADVANCED_FACE('',(#1418),#1096,.F.);
#9445=ADVANCED_FACE('',(#1419),#1097,.F.);
#9446=ADVANCED_FACE('',(#1420),#1098,.F.);
#9447=ADVANCED_FACE('',(#1421),#1099,.F.);
#9448=ADVANCED_FACE('',(#1422),#1100,.F.);
#9449=ADVANCED_FACE('',(#1423),#1101,.F.);
#9450=ADVANCED_FACE('',(#1424),#1102,.F.);
#9451=ADVANCED_FACE('',(#1425),#1103,.F.);
#9452=ADVANCED_FACE('',(#1426),#1104,.F.);
#9453=ADVANCED_FACE('',(#1427),#1105,.F.);
#9454=ADVANCED_FACE('',(#1428),#1106,.F.);
#9455=ADVANCED_FACE('',(#1429),#1107,.F.);
#9456=ADVANCED_FACE('',(#1430),#1108,.F.);
#9457=ADVANCED_FACE('',(#1431),#1109,.F.);
#9458=ADVANCED_FACE('',(#1432),#1110,.F.);
#9459=ADVANCED_FACE('',(#1433),#1111,.F.);
#9460=ADVANCED_FACE('',(#1434),#1112,.F.);
#9461=ADVANCED_FACE('',(#1435),#1113,.F.);
#9462=ADVANCED_FACE('',(#1436),#1114,.F.);
#9463=ADVANCED_FACE('',(#1437),#1115,.F.);
#9464=ADVANCED_FACE('',(#1438),#1116,.F.);
#9465=ADVANCED_FACE('',(#1439),#1117,.F.);
#9466=ADVANCED_FACE('',(#1440),#1118,.F.);
#9467=ADVANCED_FACE('',(#1441),#1119,.F.);
#9468=ADVANCED_FACE('',(#1442),#1120,.F.);
#9469=ADVANCED_FACE('',(#1443),#1121,.F.);
#9470=ADVANCED_FACE('',(#1444),#1122,.F.);
#9471=ADVANCED_FACE('',(#1445),#1123,.F.);
#9472=ADVANCED_FACE('',(#1446),#1124,.F.);
#9473=ADVANCED_FACE('',(#1447),#1125,.F.);
#9474=ADVANCED_FACE('',(#1448),#1126,.F.);
#9475=ADVANCED_FACE('',(#1449),#1127,.F.);
#9476=ADVANCED_FACE('',(#1450),#1128,.F.);
#9477=ADVANCED_FACE('',(#1451),#1129,.F.);
#9478=ADVANCED_FACE('',(#1452),#1130,.F.);
#9479=ADVANCED_FACE('',(#1453),#1131,.F.);
#9480=ADVANCED_FACE('',(#1454),#1132,.F.);
#9481=ADVANCED_FACE('',(#1455),#1133,.F.);
#9482=ADVANCED_FACE('',(#1456),#1134,.F.);
#9483=ADVANCED_FACE('',(#1457),#1135,.F.);
#9484=ADVANCED_FACE('',(#1458),#1136,.F.);
#9485=ADVANCED_FACE('',(#1459),#1137,.F.);
#9486=ADVANCED_FACE('',(#1460),#1138,.F.);
#9487=ADVANCED_FACE('',(#1461),#1139,.F.);
#9488=ADVANCED_FACE('',(#1462),#1140,.F.);
#9489=ADVANCED_FACE('',(#1463),#1141,.F.);
#9490=ADVANCED_FACE('',(#1464),#1142,.F.);
#9491=ADVANCED_FACE('',(#1465),#1143,.F.);
#9492=ADVANCED_FACE('',(#1466),#1144,.F.);
#9493=ADVANCED_FACE('',(#1467),#1145,.F.);
#9494=ADVANCED_FACE('',(#1468),#1146,.F.);
#9495=ADVANCED_FACE('',(#1469),#202,.F.);
#9496=ADVANCED_FACE('',(#1470),#1147,.T.);
#9497=ADVANCED_FACE('',(#1471),#1148,.T.);
#9498=ADVANCED_FACE('',(#1472),#1149,.T.);
#9499=ADVANCED_FACE('',(#1473),#1150,.T.);
#9500=ADVANCED_FACE('',(#1474),#1151,.T.);
#9501=ADVANCED_FACE('',(#1475),#1152,.T.);
#9502=ADVANCED_FACE('',(#1476),#1153,.T.);
#9503=ADVANCED_FACE('',(#1477),#1154,.T.);
#9504=ADVANCED_FACE('',(#1478),#1155,.T.);
#9505=ADVANCED_FACE('',(#1479),#1156,.T.);
#9506=ADVANCED_FACE('',(#1480),#1157,.T.);
#9507=ADVANCED_FACE('',(#1481),#1158,.T.);
#9508=ADVANCED_FACE('',(#1482),#1159,.T.);
#9509=ADVANCED_FACE('',(#1483),#1160,.T.);
#9510=ADVANCED_FACE('',(#1484),#1161,.T.);
#9511=ADVANCED_FACE('',(#1485),#1162,.T.);
#9512=ADVANCED_FACE('',(#1486),#1163,.T.);
#9513=ADVANCED_FACE('',(#1487),#1164,.T.);
#9514=ADVANCED_FACE('',(#1488),#1165,.T.);
#9515=ADVANCED_FACE('',(#1489),#1166,.T.);
#9516=ADVANCED_FACE('',(#1490),#1167,.T.);
#9517=ADVANCED_FACE('',(#1491),#1168,.T.);
#9518=ADVANCED_FACE('',(#1492),#1169,.T.);
#9519=ADVANCED_FACE('',(#1493),#1170,.T.);
#9520=ADVANCED_FACE('',(#1494),#1171,.T.);
#9521=ADVANCED_FACE('',(#1495),#1172,.T.);
#9522=ADVANCED_FACE('',(#1496),#1173,.T.);
#9523=ADVANCED_FACE('',(#1497),#1174,.F.);
#9524=ADVANCED_FACE('',(#1498),#1175,.T.);
#9525=ADVANCED_FACE('',(#1499),#203,.F.);
#9526=ADVANCED_FACE('',(#1500),#204,.F.);
#9527=ADVANCED_FACE('',(#1501),#1176,.T.);
#9528=ADVANCED_FACE('',(#1502),#1177,.T.);
#9529=ADVANCED_FACE('',(#1503),#1178,.T.);
#9530=ADVANCED_FACE('',(#1504),#9205,.T.);
#9531=ADVANCED_FACE('',(#1505),#9206,.T.);
#9532=ADVANCED_FACE('',(#1506,#138,#139,#140),#1179,.T.);
#9533=ADVANCED_FACE('',(#1507),#1180,.T.);
#9534=ADVANCED_FACE('',(#1508),#1181,.T.);
#9535=ADVANCED_FACE('',(#1509),#1182,.T.);
#9536=ADVANCED_FACE('',(#1510),#1183,.T.);
#9537=ADVANCED_FACE('',(#1511),#1184,.T.);
#9538=ADVANCED_FACE('',(#1512),#1185,.T.);
#9539=ADVANCED_FACE('',(#1513,#141,#142,#143),#1186,.F.);
#9890=CLOSED_SHELL('',(#9438,#9439,#9440,#9441,#9442,#9443,#9444,#9445,
#9446,#9447,#9448,#9449,#9450,#9451,#9452,#9453,#9454,#9455,#9456,#9457,
#9458,#9459,#9460,#9461,#9462,#9463,#9464,#9465,#9466,#9467,#9468,#9469,
#9470,#9471,#9472,#9473,#9474,#9475,#9476,#9477,#9478,#9479,#9480,#9481,
#9482,#9483,#9484,#9485,#9486,#9487,#9488,#9489,#9490,#9491,#9492,#9493,
#9494,#9495,#9496,#9497,#9498,#9499,#9500,#9501,#9502,#9503,#9504,#9505,
#9506,#9507,#9508,#9509,#9510,#9511,#9512,#9513,#9514,#9515,#9516,#9517,
#9518,#9519,#9520,#9521,#9522,#9523,#9524,#9525,#9526,#9527,#9528,#9529,
#9530,#9531,#9532,#9533,#9534,#9535,#9536,#9537,#9538,#9539));
#10121=AXIS2_PLACEMENT_3D('',#13734,#11017,#11018);
#10122=AXIS2_PLACEMENT_3D('',#13735,#11019,#11020);
#10123=AXIS2_PLACEMENT_3D('',#13737,#11021,#11022);
#10124=AXIS2_PLACEMENT_3D('',#13740,#11024,#11025);
#10125=AXIS2_PLACEMENT_3D('',#13741,#11026,#11027);
#10126=AXIS2_PLACEMENT_3D('',#13743,#11028,#11029);
#10127=AXIS2_PLACEMENT_3D('',#13746,#11031,#11032);
#10128=AXIS2_PLACEMENT_3D('',#13747,#11033,#11034);
#10129=AXIS2_PLACEMENT_3D('',#13749,#11035,#11036);
#10130=AXIS2_PLACEMENT_3D('',#13752,#11038,#11039);
#10131=AXIS2_PLACEMENT_3D('',#13753,#11040,#11041);
#10132=AXIS2_PLACEMENT_3D('',#13768,#11044,#11045);
#10133=AXIS2_PLACEMENT_3D('',#13780,#11047,#11048);
#10134=AXIS2_PLACEMENT_3D('',#13795,#11051,#11052);
#10135=AXIS2_PLACEMENT_3D('',#13807,#11054,#11055);
#10136=AXIS2_PLACEMENT_3D('',#13822,#11058,#11059);
#10137=AXIS2_PLACEMENT_3D('',#13834,#11061,#11062);
#10138=AXIS2_PLACEMENT_3D('',#13849,#11065,#11066);
#10139=AXIS2_PLACEMENT_3D('',#13861,#11068,#11069);
#10140=AXIS2_PLACEMENT_3D('',#13876,#11072,#11073);
#10141=AXIS2_PLACEMENT_3D('',#13888,#11075,#11076);
#10142=AXIS2_PLACEMENT_3D('',#13903,#11079,#11080);
#10143=AXIS2_PLACEMENT_3D('',#13915,#11082,#11083);
#10144=AXIS2_PLACEMENT_3D('',#13930,#11086,#11087);
#10145=AXIS2_PLACEMENT_3D('',#13942,#11089,#11090);
#10146=AXIS2_PLACEMENT_3D('',#13957,#11093,#11094);
#10147=AXIS2_PLACEMENT_3D('',#13969,#11096,#11097);
#10148=AXIS2_PLACEMENT_3D('',#13984,#11100,#11101);
#10149=AXIS2_PLACEMENT_3D('',#13996,#11103,#11104);
#10150=AXIS2_PLACEMENT_3D('',#14011,#11107,#11108);
#10151=AXIS2_PLACEMENT_3D('',#14023,#11110,#11111);
#10152=AXIS2_PLACEMENT_3D('',#14038,#11114,#11115);
#10153=AXIS2_PLACEMENT_3D('',#14050,#11117,#11118);
#10154=AXIS2_PLACEMENT_3D('',#14065,#11121,#11122);
#10155=AXIS2_PLACEMENT_3D('',#14077,#11124,#11125);
#10156=AXIS2_PLACEMENT_3D('',#14092,#11128,#11129);
#10157=AXIS2_PLACEMENT_3D('',#14104,#11131,#11132);
#10158=AXIS2_PLACEMENT_3D('',#14119,#11135,#11136);
#10159=AXIS2_PLACEMENT_3D('',#14131,#11138,#11139);
#10160=AXIS2_PLACEMENT_3D('',#14146,#11142,#11143);
#10161=AXIS2_PLACEMENT_3D('',#14158,#11145,#11146);
#10162=AXIS2_PLACEMENT_3D('',#14173,#11149,#11150);
#10163=AXIS2_PLACEMENT_3D('',#14185,#11152,#11153);
#10164=AXIS2_PLACEMENT_3D('',#14200,#11156,#11157);
#10165=AXIS2_PLACEMENT_3D('',#14212,#11159,#11160);
#10166=AXIS2_PLACEMENT_3D('',#14227,#11163,#11164);
#10167=AXIS2_PLACEMENT_3D('',#14239,#11166,#11167);
#10168=AXIS2_PLACEMENT_3D('',#14254,#11170,#11171);
#10169=AXIS2_PLACEMENT_3D('',#14266,#11173,#11174);
#10170=AXIS2_PLACEMENT_3D('',#14281,#11177,#11178);
#10171=AXIS2_PLACEMENT_3D('',#14293,#11180,#11181);
#10172=AXIS2_PLACEMENT_3D('',#14308,#11184,#11185);
#10173=AXIS2_PLACEMENT_3D('',#14320,#11187,#11188);
#10174=AXIS2_PLACEMENT_3D('',#14335,#11191,#11192);
#10175=AXIS2_PLACEMENT_3D('',#14347,#11194,#11195);
#10176=AXIS2_PLACEMENT_3D('',#14362,#11198,#11199);
#10177=AXIS2_PLACEMENT_3D('',#14374,#11201,#11202);
#10178=AXIS2_PLACEMENT_3D('',#14389,#11205,#11206);
#10179=AXIS2_PLACEMENT_3D('',#14401,#11208,#11209);
#10180=AXIS2_PLACEMENT_3D('',#14416,#11212,#11213);
#10181=AXIS2_PLACEMENT_3D('',#14428,#11215,#11216);
#10182=AXIS2_PLACEMENT_3D('',#14443,#11219,#11220);
#10183=AXIS2_PLACEMENT_3D('',#14455,#11222,#11223);
#10184=AXIS2_PLACEMENT_3D('',#14470,#11226,#11227);
#10185=AXIS2_PLACEMENT_3D('',#14622,#11231,#11232);
#10186=AXIS2_PLACEMENT_3D('',#14629,#11234,#11235);
#10187=AXIS2_PLACEMENT_3D('',#14642,#11240,#11241);
#10188=AXIS2_PLACEMENT_3D('',#14647,#11242,#11243);
#10189=AXIS2_PLACEMENT_3D('',#14652,#11244,#11245);
#10190=AXIS2_PLACEMENT_3D('',#14657,#11246,#11247);
#10191=AXIS2_PLACEMENT_3D('',#14662,#11248,#11249);
#10192=AXIS2_PLACEMENT_3D('',#14667,#11250,#11251);
#10193=AXIS2_PLACEMENT_3D('',#14672,#11252,#11253);
#10194=AXIS2_PLACEMENT_3D('',#14677,#11254,#11255);
#10195=AXIS2_PLACEMENT_3D('',#14682,#11256,#11257);
#10196=AXIS2_PLACEMENT_3D('',#14687,#11258,#11259);
#10197=AXIS2_PLACEMENT_3D('',#14692,#11260,#11261);
#10198=AXIS2_PLACEMENT_3D('',#14697,#11262,#11263);
#10199=AXIS2_PLACEMENT_3D('',#14702,#11264,#11265);
#10200=AXIS2_PLACEMENT_3D('',#14707,#11266,#11267);
#10201=AXIS2_PLACEMENT_3D('',#14712,#11268,#11269);
#10202=AXIS2_PLACEMENT_3D('',#14717,#11270,#11271);
#10203=AXIS2_PLACEMENT_3D('',#14722,#11272,#11273);
#10204=AXIS2_PLACEMENT_3D('',#14727,#11274,#11275);
#10205=AXIS2_PLACEMENT_3D('',#14732,#11276,#11277);
#10206=AXIS2_PLACEMENT_3D('',#14737,#11278,#11279);
#10207=AXIS2_PLACEMENT_3D('',#14742,#11280,#11281);
#10208=AXIS2_PLACEMENT_3D('',#14747,#11282,#11283);
#10209=AXIS2_PLACEMENT_3D('',#14752,#11284,#11285);
#10210=AXIS2_PLACEMENT_3D('',#14757,#11286,#11287);
#10211=AXIS2_PLACEMENT_3D('',#14762,#11288,#11289);
#10212=AXIS2_PLACEMENT_3D('',#14767,#11290,#11291);
#10213=AXIS2_PLACEMENT_3D('',#14771,#11294,#11295);
#10214=AXIS2_PLACEMENT_3D('',#14820,#11300,#11301);
#10215=AXIS2_PLACEMENT_3D('',#14821,#11302,#11303);
#10216=AXIS2_PLACEMENT_3D('',#14827,#11307,#11308);
#10217=AXIS2_PLACEMENT_3D('',#14833,#11312,#11313);
#10218=AXIS2_PLACEMENT_3D('',#14835,#11314,#11315);
#10219=AXIS2_PLACEMENT_3D('',#14838,#11317,#11318);
#10220=AXIS2_PLACEMENT_3D('',#14839,#11319,#11320);
#10221=AXIS2_PLACEMENT_3D('',#14841,#11321,#11322);
#10222=AXIS2_PLACEMENT_3D('',#14844,#11324,#11325);
#10223=AXIS2_PLACEMENT_3D('',#14845,#11326,#11327);
#10224=AXIS2_PLACEMENT_3D('',#14857,#11334,#11335);
#10225=AXIS2_PLACEMENT_3D('',#14861,#11338,#11339);
#10226=AXIS2_PLACEMENT_3D('',#14865,#11342,#11343);
#10227=AXIS2_PLACEMENT_3D('',#14869,#11346,#11347);
#10228=AXIS2_PLACEMENT_3D('',#14873,#11350,#11351);
#10229=AXIS2_PLACEMENT_3D('',#14877,#11354,#11355);
#10230=AXIS2_PLACEMENT_3D('',#14879,#11357,#11358);
#11017=DIRECTION('axis',(0.,0.,1.));
#11018=DIRECTION('refdir',(1.,0.,0.));
#11019=DIRECTION('center_axis',(0.,0.,-1.));
#11020=DIRECTION('ref_axis',(1.,0.,0.));
#11021=DIRECTION('center_axis',(0.,0.,-1.));
#11022=DIRECTION('ref_axis',(1.,0.,0.));
#11023=DIRECTION('',(0.,0.,-1.));
#11024=DIRECTION('center_axis',(0.,0.,1.));
#11025=DIRECTION('ref_axis',(1.,0.,0.));
#11026=DIRECTION('center_axis',(0.,0.,-1.));
#11027=DIRECTION('ref_axis',(1.,0.,0.));
#11028=DIRECTION('center_axis',(0.,0.,-1.));
#11029=DIRECTION('ref_axis',(1.,0.,0.));
#11030=DIRECTION('',(0.,0.,-1.));
#11031=DIRECTION('center_axis',(0.,0.,1.));
#11032=DIRECTION('ref_axis',(1.,0.,0.));
#11033=DIRECTION('center_axis',(0.,0.,-1.));
#11034=DIRECTION('ref_axis',(1.,0.,0.));
#11035=DIRECTION('center_axis',(0.,0.,-1.));
#11036=DIRECTION('ref_axis',(1.,0.,0.));
#11037=DIRECTION('',(0.,0.,-1.));
#11038=DIRECTION('center_axis',(0.,0.,1.));
#11039=DIRECTION('ref_axis',(1.,0.,0.));
#11040=DIRECTION('center_axis',(-0.776114000116266,0.630592625094466,0.));
#11041=DIRECTION('ref_axis',(0.630592625094466,0.776114000116266,0.));
#11042=DIRECTION('',(0.,0.,-1.));
#11043=DIRECTION('',(0.,0.,1.));
#11044=DIRECTION('center_axis',(0.776114000116266,0.630592625094466,0.));
#11045=DIRECTION('ref_axis',(0.630592625094466,-0.776114000116266,0.));
#11046=DIRECTION('',(0.,0.,-1.));
#11047=DIRECTION('center_axis',(-0.776114000116266,0.630592625094466,0.));
#11048=DIRECTION('ref_axis',(0.630592625094466,0.776114000116266,0.));
#11049=DIRECTION('',(0.,0.,-1.));
#11050=DIRECTION('',(0.,0.,1.));
#11051=DIRECTION('center_axis',(0.776114000116268,0.630592625094463,0.));
#11052=DIRECTION('ref_axis',(0.630592625094463,-0.776114000116268,0.));
#11053=DIRECTION('',(0.,0.,-1.));
#11054=DIRECTION('center_axis',(-0.776114000116268,0.630592625094463,0.));
#11055=DIRECTION('ref_axis',(0.630592625094463,0.776114000116268,0.));
#11056=DIRECTION('',(0.,0.,-1.));
#11057=DIRECTION('',(0.,0.,1.));
#11058=DIRECTION('center_axis',(0.776114000116266,0.630592625094466,0.));
#11059=DIRECTION('ref_axis',(0.630592625094466,-0.776114000116266,0.));
#11060=DIRECTION('',(0.,0.,-1.));
#11061=DIRECTION('center_axis',(-0.776114000116264,0.630592625094468,0.));
#11062=DIRECTION('ref_axis',(0.630592625094468,0.776114000116264,0.));
#11063=DIRECTION('',(0.,0.,-1.));
#11064=DIRECTION('',(0.,0.,1.));
#11065=DIRECTION('center_axis',(0.776114000116268,0.630592625094463,0.));
#11066=DIRECTION('ref_axis',(0.630592625094463,-0.776114000116268,0.));
#11067=DIRECTION('',(0.,0.,-1.));
#11068=DIRECTION('center_axis',(-0.776114000116268,0.630592625094463,0.));
#11069=DIRECTION('ref_axis',(0.630592625094463,0.776114000116268,0.));
#11070=DIRECTION('',(0.,0.,-1.));
#11071=DIRECTION('',(0.,0.,1.));
#11072=DIRECTION('center_axis',(0.776114000116268,0.630592625094463,0.));
#11073=DIRECTION('ref_axis',(0.630592625094463,-0.776114000116268,0.));
#11074=DIRECTION('',(0.,0.,-1.));
#11075=DIRECTION('center_axis',(-0.776114000116268,0.630592625094463,0.));
#11076=DIRECTION('ref_axis',(0.630592625094463,0.776114000116268,0.));
#11077=DIRECTION('',(0.,0.,-1.));
#11078=DIRECTION('',(0.,0.,1.));
#11079=DIRECTION('center_axis',(0.776114000116264,0.630592625094468,0.));
#11080=DIRECTION('ref_axis',(0.630592625094468,-0.776114000116264,0.));
#11081=DIRECTION('',(0.,0.,-1.));
#11082=DIRECTION('center_axis',(-0.776114000116264,0.630592625094468,0.));
#11083=DIRECTION('ref_axis',(0.630592625094468,0.776114000116264,0.));
#11084=DIRECTION('',(0.,0.,-1.));
#11085=DIRECTION('',(0.,0.,1.));
#11086=DIRECTION('center_axis',(0.776114000116259,0.630592625094473,0.));
#11087=DIRECTION('ref_axis',(0.630592625094473,-0.776114000116259,0.));
#11088=DIRECTION('',(0.,0.,-1.));
#11089=DIRECTION('center_axis',(-0.776114000116268,0.630592625094463,0.));
#11090=DIRECTION('ref_axis',(0.630592625094463,0.776114000116268,0.));
#11091=DIRECTION('',(0.,0.,-1.));
#11092=DIRECTION('',(0.,0.,1.));
#11093=DIRECTION('center_axis',(0.776114000116268,0.630592625094463,0.));
#11094=DIRECTION('ref_axis',(0.630592625094463,-0.776114000116268,0.));
#11095=DIRECTION('',(0.,0.,-1.));
#11096=DIRECTION('center_axis',(-0.776114000116268,0.630592625094463,0.));
#11097=DIRECTION('ref_axis',(0.630592625094463,0.776114000116268,0.));
#11098=DIRECTION('',(0.,0.,-1.));
#11099=DIRECTION('',(0.,0.,1.));
#11100=DIRECTION('center_axis',(0.776114000116264,0.630592625094468,0.));
#11101=DIRECTION('ref_axis',(0.630592625094468,-0.776114000116264,0.));
#11102=DIRECTION('',(0.,0.,-1.));
#11103=DIRECTION('center_axis',(-0.776114000116264,0.630592625094468,0.));
#11104=DIRECTION('ref_axis',(0.630592625094468,0.776114000116264,0.));
#11105=DIRECTION('',(0.,0.,-1.));
#11106=DIRECTION('',(0.,0.,1.));
#11107=DIRECTION('center_axis',(0.776114000116268,0.630592625094463,0.));
#11108=DIRECTION('ref_axis',(0.630592625094463,-0.776114000116268,0.));
#11109=DIRECTION('',(0.,0.,-1.));
#11110=DIRECTION('center_axis',(-0.776114000116264,0.630592625094468,0.));
#11111=DIRECTION('ref_axis',(0.630592625094468,0.776114000116264,0.));
#11112=DIRECTION('',(0.,0.,-1.));
#11113=DIRECTION('',(0.,0.,1.));
#11114=DIRECTION('center_axis',(0.776114000116264,0.630592625094468,0.));
#11115=DIRECTION('ref_axis',(0.630592625094468,-0.776114000116264,0.));
#11116=DIRECTION('',(0.,0.,-1.));
#11117=DIRECTION('center_axis',(-0.776114000116259,0.630592625094473,0.));
#11118=DIRECTION('ref_axis',(0.630592625094473,0.776114000116259,0.));
#11119=DIRECTION('',(0.,0.,-1.));
#11120=DIRECTION('',(0.,0.,1.));
#11121=DIRECTION('center_axis',(0.776114000116264,0.630592625094468,0.));
#11122=DIRECTION('ref_axis',(0.630592625094468,-0.776114000116264,0.));
#11123=DIRECTION('',(0.,0.,-1.));
#11124=DIRECTION('center_axis',(-0.776114000116264,0.630592625094468,0.));
#11125=DIRECTION('ref_axis',(0.630592625094468,0.776114000116264,0.));
#11126=DIRECTION('',(0.,0.,-1.));
#11127=DIRECTION('',(0.,0.,1.));
#11128=DIRECTION('center_axis',(0.776114000116264,0.630592625094468,0.));
#11129=DIRECTION('ref_axis',(0.630592625094468,-0.776114000116264,0.));
#11130=DIRECTION('',(0.,0.,-1.));
#11131=DIRECTION('center_axis',(-0.776114000116264,0.630592625094468,0.));
#11132=DIRECTION('ref_axis',(0.630592625094468,0.776114000116264,0.));
#11133=DIRECTION('',(0.,0.,-1.));
#11134=DIRECTION('',(0.,0.,1.));
#11135=DIRECTION('center_axis',(0.776114000116264,0.630592625094468,0.));
#11136=DIRECTION('ref_axis',(0.630592625094468,-0.776114000116264,0.));
#11137=DIRECTION('',(0.,0.,-1.));
#11138=DIRECTION('center_axis',(-0.776114000116264,0.630592625094468,0.));
#11139=DIRECTION('ref_axis',(0.630592625094468,0.776114000116264,0.));
#11140=DIRECTION('',(0.,0.,-1.));
#11141=DIRECTION('',(0.,0.,1.));
#11142=DIRECTION('center_axis',(0.776114000116264,0.630592625094468,0.));
#11143=DIRECTION('ref_axis',(0.630592625094468,-0.776114000116264,0.));
#11144=DIRECTION('',(0.,0.,-1.));
#11145=DIRECTION('center_axis',(-0.776114000116264,0.630592625094468,0.));
#11146=DIRECTION('ref_axis',(0.630592625094468,0.776114000116264,0.));
#11147=DIRECTION('',(0.,0.,-1.));
#11148=DIRECTION('',(0.,0.,1.));
#11149=DIRECTION('center_axis',(0.776114000116259,0.630592625094473,0.));
#11150=DIRECTION('ref_axis',(0.630592625094473,-0.776114000116259,0.));
#11151=DIRECTION('',(0.,0.,-1.));
#11152=DIRECTION('center_axis',(-0.776114000116264,0.630592625094468,0.));
#11153=DIRECTION('ref_axis',(0.630592625094468,0.776114000116264,0.));
#11154=DIRECTION('',(0.,0.,-1.));
#11155=DIRECTION('',(0.,0.,1.));
#11156=DIRECTION('center_axis',(0.776114000116264,0.630592625094468,0.));
#11157=DIRECTION('ref_axis',(0.630592625094468,-0.776114000116264,0.));
#11158=DIRECTION('',(0.,0.,-1.));
#11159=DIRECTION('center_axis',(-0.776114000116264,0.630592625094468,0.));
#11160=DIRECTION('ref_axis',(0.630592625094468,0.776114000116264,0.));
#11161=DIRECTION('',(0.,0.,-1.));
#11162=DIRECTION('',(0.,0.,1.));
#11163=DIRECTION('center_axis',(0.776114000116268,0.630592625094463,0.));
#11164=DIRECTION('ref_axis',(0.630592625094463,-0.776114000116268,0.));
#11165=DIRECTION('',(0.,0.,-1.));
#11166=DIRECTION('center_axis',(-0.776114000116268,0.630592625094463,0.));
#11167=DIRECTION('ref_axis',(0.630592625094463,0.776114000116268,0.));
#11168=DIRECTION('',(0.,0.,-1.));
#11169=DIRECTION('',(0.,0.,1.));
#11170=DIRECTION('center_axis',(0.776114000116264,0.630592625094468,0.));
#11171=DIRECTION('ref_axis',(0.630592625094468,-0.776114000116264,0.));
#11172=DIRECTION('',(0.,0.,-1.));
#11173=DIRECTION('center_axis',(-0.776114000116264,0.630592625094468,0.));
#11174=DIRECTION('ref_axis',(0.630592625094468,0.776114000116264,0.));
#11175=DIRECTION('',(0.,0.,-1.));
#11176=DIRECTION('',(0.,0.,1.));
#11177=DIRECTION('center_axis',(0.776114000116268,0.630592625094463,0.));
#11178=DIRECTION('ref_axis',(0.630592625094463,-0.776114000116268,0.));
#11179=DIRECTION('',(0.,0.,-1.));
#11180=DIRECTION('center_axis',(-0.776114000116264,0.630592625094468,0.));
#11181=DIRECTION('ref_axis',(0.630592625094468,0.776114000116264,0.));
#11182=DIRECTION('',(0.,0.,-1.));
#11183=DIRECTION('',(0.,0.,1.));
#11184=DIRECTION('center_axis',(0.776114000116268,0.630592625094463,0.));
#11185=DIRECTION('ref_axis',(0.630592625094463,-0.776114000116268,0.));
#11186=DIRECTION('',(0.,0.,-1.));
#11187=DIRECTION('center_axis',(-0.776114000116268,0.630592625094463,0.));
#11188=DIRECTION('ref_axis',(0.630592625094463,0.776114000116268,0.));
#11189=DIRECTION('',(0.,0.,-1.));
#11190=DIRECTION('',(0.,0.,1.));
#11191=DIRECTION('center_axis',(0.776114000116264,0.630592625094468,0.));
#11192=DIRECTION('ref_axis',(0.630592625094468,-0.776114000116264,0.));
#11193=DIRECTION('',(0.,0.,-1.));
#11194=DIRECTION('center_axis',(-0.776114000116264,0.630592625094468,0.));
#11195=DIRECTION('ref_axis',(0.630592625094468,0.776114000116264,0.));
#11196=DIRECTION('',(0.,0.,-1.));
#11197=DIRECTION('',(0.,0.,1.));
#11198=DIRECTION('center_axis',(0.776114000116268,0.630592625094463,0.));
#11199=DIRECTION('ref_axis',(0.630592625094463,-0.776114000116268,0.));
#11200=DIRECTION('',(0.,0.,-1.));
#11201=DIRECTION('center_axis',(-0.776114000116266,0.630592625094466,0.));
#11202=DIRECTION('ref_axis',(0.630592625094466,0.776114000116266,0.));
#11203=DIRECTION('',(0.,0.,-1.));
#11204=DIRECTION('',(0.,0.,1.));
#11205=DIRECTION('center_axis',(0.776114000116266,0.630592625094466,0.));
#11206=DIRECTION('ref_axis',(0.630592625094466,-0.776114000116266,0.));
#11207=DIRECTION('',(0.,0.,-1.));
#11208=DIRECTION('center_axis',(-0.776114000116266,0.630592625094466,0.));
#11209=DIRECTION('ref_axis',(0.630592625094466,0.776114000116266,0.));
#11210=DIRECTION('',(0.,0.,-1.));
#11211=DIRECTION('',(0.,0.,1.));
#11212=DIRECTION('center_axis',(0.776114000116266,0.630592625094466,0.));
#11213=DIRECTION('ref_axis',(0.630592625094466,-0.776114000116266,0.));
#11214=DIRECTION('',(0.,0.,-1.));
#11215=DIRECTION('center_axis',(-0.776114000116266,0.630592625094466,0.));
#11216=DIRECTION('ref_axis',(0.630592625094466,0.776114000116266,0.));
#11217=DIRECTION('',(0.,0.,-1.));
#11218=DIRECTION('',(0.,0.,1.));
#11219=DIRECTION('center_axis',(0.776114000116266,0.630592625094466,0.));
#11220=DIRECTION('ref_axis',(0.630592625094466,-0.776114000116266,0.));
#11221=DIRECTION('',(0.,0.,-1.));
#11222=DIRECTION('center_axis',(-0.776114000116268,0.630592625094463,0.));
#11223=DIRECTION('ref_axis',(0.630592625094463,0.776114000116268,0.));
#11224=DIRECTION('',(0.,0.,-1.));
#11225=DIRECTION('',(0.,0.,1.));
#11226=DIRECTION('center_axis',(0.776114000116266,0.630592625094466,0.));
#11227=DIRECTION('ref_axis',(0.630592625094466,-0.776114000116266,0.));
#11228=DIRECTION('',(0.,0.,-1.));
#11229=DIRECTION('',(0.,1.,0.));
#11230=DIRECTION('',(0.,1.,0.));
#11231=DIRECTION('center_axis',(0.,-1.,0.));
#11232=DIRECTION('ref_axis',(1.,0.,0.));
#11233=DIRECTION('',(0.,0.,-1.));
#11234=DIRECTION('center_axis',(0.,-1.,0.));
#11235=DIRECTION('ref_axis',(1.,0.,0.));
#11236=DIRECTION('',(0.,0.,-1.));
#11237=DIRECTION('',(-1.,0.,0.));
#11238=DIRECTION('',(0.,0.,-1.));
#11239=DIRECTION('',(1.,0.,0.));
#11240=DIRECTION('center_axis',(0.,-1.,0.));
#11241=DIRECTION('ref_axis',(1.,0.,0.));
#11242=DIRECTION('center_axis',(0.,-1.,0.));
#11243=DIRECTION('ref_axis',(1.,0.,0.));
#11244=DIRECTION('center_axis',(0.,-1.,0.));
#11245=DIRECTION('ref_axis',(1.,0.,0.));
#11246=DIRECTION('center_axis',(0.,-1.,0.));
#11247=DIRECTION('ref_axis',(1.,0.,0.));
#11248=DIRECTION('center_axis',(0.,-1.,0.));
#11249=DIRECTION('ref_axis',(1.,0.,0.));
#11250=DIRECTION('center_axis',(0.,-1.,0.));
#11251=DIRECTION('ref_axis',(1.,0.,0.));
#11252=DIRECTION('center_axis',(0.,-1.,0.));
#11253=DIRECTION('ref_axis',(1.,0.,0.));
#11254=DIRECTION('center_axis',(0.,-1.,0.));
#11255=DIRECTION('ref_axis',(1.,0.,0.));
#11256=DIRECTION('center_axis',(0.,-1.,0.));
#11257=DIRECTION('ref_axis',(1.,0.,0.));
#11258=DIRECTION('center_axis',(0.,-1.,0.));
#11259=DIRECTION('ref_axis',(1.,0.,0.));
#11260=DIRECTION('center_axis',(0.,-1.,0.));
#11261=DIRECTION('ref_axis',(1.,0.,0.));
#11262=DIRECTION('center_axis',(0.,-1.,0.));
#11263=DIRECTION('ref_axis',(1.,0.,0.));
#11264=DIRECTION('center_axis',(0.,-1.,0.));
#11265=DIRECTION('ref_axis',(1.,0.,0.));
#11266=DIRECTION('center_axis',(0.,-1.,0.));
#11267=DIRECTION('ref_axis',(1.,0.,0.));
#11268=DIRECTION('center_axis',(0.,-1.,0.));
#11269=DIRECTION('ref_axis',(1.,0.,0.));
#11270=DIRECTION('center_axis',(0.,-1.,0.));
#11271=DIRECTION('ref_axis',(1.,0.,0.));
#11272=DIRECTION('center_axis',(0.,-1.,0.));
#11273=DIRECTION('ref_axis',(1.,0.,0.));
#11274=DIRECTION('center_axis',(0.,-1.,0.));
#11275=DIRECTION('ref_axis',(1.,0.,0.));
#11276=DIRECTION('center_axis',(0.,-1.,0.));
#11277=DIRECTION('ref_axis',(1.,0.,0.));
#11278=DIRECTION('center_axis',(0.,-1.,0.));
#11279=DIRECTION('ref_axis',(1.,0.,0.));
#11280=DIRECTION('center_axis',(0.,-1.,0.));
#11281=DIRECTION('ref_axis',(1.,0.,0.));
#11282=DIRECTION('center_axis',(0.,-1.,0.));
#11283=DIRECTION('ref_axis',(1.,0.,0.));
#11284=DIRECTION('center_axis',(0.,-1.,0.));
#11285=DIRECTION('ref_axis',(1.,0.,0.));
#11286=DIRECTION('center_axis',(0.,-1.,0.));
#11287=DIRECTION('ref_axis',(1.,0.,0.));
#11288=DIRECTION('center_axis',(0.,-1.,0.));
#11289=DIRECTION('ref_axis',(1.,0.,0.));
#11290=DIRECTION('center_axis',(1.,-4.12091517652768E-29,3.50314129644857E-29));
#11291=DIRECTION('ref_axis',(3.50314129644857E-29,0.,-1.));
#11292=DIRECTION('',(0.,-1.,0.));
#11293=DIRECTION('',(0.,0.,1.));
#11294=DIRECTION('center_axis',(1.,0.,0.));
#11295=DIRECTION('ref_axis',(0.,0.,-1.));
#11296=DIRECTION('',(0.,1.,0.));
#11297=DIRECTION('',(0.,0.,1.));
#11298=DIRECTION('',(0.,0.,1.));
#11299=DIRECTION('',(0.,-1.,0.));
#11300=DIRECTION('center_axis',(0.,-1.,0.));
#11301=DIRECTION('ref_axis',(1.,0.,0.));
#11302=DIRECTION('center_axis',(0.,1.,0.));
#11303=DIRECTION('ref_axis',(-1.,0.,0.));
#11304=DIRECTION('',(1.,0.,0.));
#11305=DIRECTION('',(-1.,0.,0.));
#11306=DIRECTION('',(0.,0.,1.));
#11307=DIRECTION('center_axis',(1.,0.,0.));
#11308=DIRECTION('ref_axis',(0.,1.,0.));
#11309=DIRECTION('',(0.,0.,1.));
#11310=DIRECTION('',(0.,-1.,0.));
#11311=DIRECTION('',(0.,1.,0.));
#11312=DIRECTION('center_axis',(0.,0.,1.));
#11313=DIRECTION('ref_axis',(1.,0.,0.));
#11314=DIRECTION('center_axis',(0.,0.,1.));
#11315=DIRECTION('ref_axis',(1.,0.,0.));
#11316=DIRECTION('',(0.,0.,1.));
#11317=DIRECTION('center_axis',(0.,0.,1.));
#11318=DIRECTION('ref_axis',(1.,0.,0.));
#11319=DIRECTION('center_axis',(0.,0.,1.));
#11320=DIRECTION('ref_axis',(1.,0.,0.));
#11321=DIRECTION('center_axis',(0.,0.,1.));
#11322=DIRECTION('ref_axis',(1.,0.,0.));
#11323=DIRECTION('',(0.,0.,-1.));
#11324=DIRECTION('center_axis',(0.,0.,1.));
#11325=DIRECTION('ref_axis',(1.,0.,0.));
#11326=DIRECTION('center_axis',(0.,0.,1.));
#11327=DIRECTION('ref_axis',(1.,0.,0.));
#11328=DIRECTION('',(0.87524153543927,-0.483686111690123,0.));
#11329=DIRECTION('',(1.,0.,0.));
#11330=DIRECTION('',(0.,1.,0.));
#11331=DIRECTION('',(-1.,0.,0.));
#11332=DIRECTION('',(-0.694594513699567,0.719401460617409,0.));
#11333=DIRECTION('',(-0.447213595499958,-0.894427190999916,0.));
#11334=DIRECTION('center_axis',(-0.483686111690123,-0.87524153543927,0.));
#11335=DIRECTION('ref_axis',(0.87524153543927,-0.483686111690123,0.));
#11336=DIRECTION('',(0.87524153543927,-0.483686111690123,0.));
#11337=DIRECTION('',(0.,0.,1.));
#11338=DIRECTION('center_axis',(-0.894427190999916,0.447213595499958,0.));
#11339=DIRECTION('ref_axis',(-0.447213595499958,-0.894427190999916,0.));
#11340=DIRECTION('',(0.,0.,1.));
#11341=DIRECTION('',(-0.447213595499958,-0.894427190999916,0.));
#11342=DIRECTION('center_axis',(0.719401460617409,0.694594513699567,0.));
#11343=DIRECTION('ref_axis',(-0.694594513699567,0.719401460617409,0.));
#11344=DIRECTION('',(-0.694594513699567,0.719401460617409,0.));
#11345=DIRECTION('',(0.,0.,1.));
#11346=DIRECTION('center_axis',(0.,1.,0.));
#11347=DIRECTION('ref_axis',(-1.,0.,0.));
#11348=DIRECTION('',(-1.,0.,0.));
#11349=DIRECTION('',(0.,0.,1.));
#11350=DIRECTION('center_axis',(1.,0.,0.));
#11351=DIRECTION('ref_axis',(0.,1.,0.));
#11352=DIRECTION('',(0.,1.,0.));
#11353=DIRECTION('',(0.,0.,1.));
#11354=DIRECTION('center_axis',(0.,-1.,0.));
#11355=DIRECTION('ref_axis',(1.,0.,0.));
#11356=DIRECTION('',(1.,0.,0.));
#11357=DIRECTION('center_axis',(0.,0.,1.));
#11358=DIRECTION('ref_axis',(1.,0.,0.));
#13734=CARTESIAN_POINT('',(0.,0.,0.));
#13735=CARTESIAN_POINT('Origin',(6.,-2.5,0.3));
#13736=CARTESIAN_POINT('',(5.83,-2.5,0.6));
#13737=CARTESIAN_POINT('Origin',(6.,-2.5,0.6));
#13738=CARTESIAN_POINT('',(5.83,-2.5,0.));
#13739=CARTESIAN_POINT('',(5.83,-2.5,0.3));
#13740=CARTESIAN_POINT('Origin',(6.,-2.5,0.));
#13741=CARTESIAN_POINT('Origin',(12.8,-2.5,0.3));
#13742=CARTESIAN_POINT('',(12.63,-2.5,0.6));
#13743=CARTESIAN_POINT('Origin',(12.8,-2.5,0.6));
#13744=CARTESIAN_POINT('',(12.63,-2.5,0.));
#13745=CARTESIAN_POINT('',(12.63,-2.5,0.3));
#13746=CARTESIAN_POINT('Origin',(12.8,-2.5,0.));
#13747=CARTESIAN_POINT('Origin',(0.,0.,0.3));
#13748=CARTESIAN_POINT('',(-0.41,5.02105187650415E-17,0.6));
#13749=CARTESIAN_POINT('Origin',(0.,0.,0.6));
#13750=CARTESIAN_POINT('',(-0.41,5.02105187650415E-17,0.));
#13751=CARTESIAN_POINT('',(-0.41,5.02105187650415E-17,0.3));
#13752=CARTESIAN_POINT('Origin',(0.,0.,0.));
#13753=CARTESIAN_POINT('Origin',(-2.965,-0.01,3.));
#13754=CARTESIAN_POINT('',(-2.9,0.07,-0.106801782385477));
#13755=CARTESIAN_POINT('',(-2.956875,4.02009657719485E-17,-0.0984757719280371));
#13756=CARTESIAN_POINT('Ctrl Pts',(-2.9,0.07,-0.106801782385477));
#13757=CARTESIAN_POINT('Ctrl Pts',(-2.91895366237794,0.0466724155348489,
-0.103946669053578));
#13758=CARTESIAN_POINT('Ctrl Pts',(-2.93791212006184,0.023338929154658,
-0.101171036891752));
#13759=CARTESIAN_POINT('Ctrl Pts',(-2.956875,0.,-0.0984757719280371));
#13760=CARTESIAN_POINT('',(-2.9,0.07,0.793198217614523));
#13761=CARTESIAN_POINT('',(-2.9,0.07,3.));
#13762=CARTESIAN_POINT('',(-2.956875,1.25075529674416E-16,0.801524228071963));
#13763=CARTESIAN_POINT('Ctrl Pts',(-2.956875,1.05932212640155E-16,0.801524228071963));
#13764=CARTESIAN_POINT('Ctrl Pts',(-2.93791212006163,0.0233389291549168,
0.798828963108218));
#13765=CARTESIAN_POINT('Ctrl Pts',(-2.91895366237815,0.0466724155345894,
0.796053330946456));
#13766=CARTESIAN_POINT('Ctrl Pts',(-2.9,0.07,0.793198217614523));
#13767=CARTESIAN_POINT('',(-2.956875,2.77555756156289E-17,1.5));
#13768=CARTESIAN_POINT('Origin',(-2.9,0.07,3.));
#13769=CARTESIAN_POINT('',(-2.843125,4.37561532211684E-17,-0.115609256379697));
#13770=CARTESIAN_POINT('Ctrl Pts',(-2.843125,0.,-0.115609256379697));
#13771=CARTESIAN_POINT('Ctrl Pts',(-2.86207835453579,0.0233272055825088,
-0.112594450424136));
#13772=CARTESIAN_POINT('Ctrl Pts',(-2.88103681218866,0.0466606919245074,
-0.109658330595625));
#13773=CARTESIAN_POINT('Ctrl Pts',(-2.9,0.07,-0.106801782385477));
#13774=CARTESIAN_POINT('',(-2.843125,9.54610500790436E-18,0.784390743620303));
#13775=CARTESIAN_POINT('',(-2.843125,-2.77555756156289E-17,1.5));
#13776=CARTESIAN_POINT('Ctrl Pts',(-2.9,0.07,0.793198217614523));
#13777=CARTESIAN_POINT('Ctrl Pts',(-2.88103681218888,0.0466606919247747,
0.790341669404405));
#13778=CARTESIAN_POINT('Ctrl Pts',(-2.86207835453559,0.0233272055822619,
0.787405549575833));
#13779=CARTESIAN_POINT('Ctrl Pts',(-2.843125,9.48706037891828E-17,0.784390743620303));
#13780=CARTESIAN_POINT('Origin',(-3.365,-0.01,3.));
#13781=CARTESIAN_POINT('',(-3.3,0.07,-0.058707352173212));
#13782=CARTESIAN_POINT('',(-3.356875,4.02009657719485E-17,-0.0538921790467937));
#13783=CARTESIAN_POINT('Ctrl Pts',(-3.3,0.07,-0.058707352173212));
#13784=CARTESIAN_POINT('Ctrl Pts',(-3.31895541554317,0.0466702577930196,
-0.0570167934636838));
#13785=CARTESIAN_POINT('Ctrl Pts',(-3.33791387480007,0.0233367694768411,
-0.0554114346567312));
#13786=CARTESIAN_POINT('Ctrl Pts',(-3.356875,0.,-0.0538921790467937));
#13787=CARTESIAN_POINT('',(-3.3,0.07,0.841292647826788));
#13788=CARTESIAN_POINT('',(-3.3,0.07,3.));
#13789=CARTESIAN_POINT('',(-3.356875,1.5362076984536E-16,0.846107820953206));
#13790=CARTESIAN_POINT('Ctrl Pts',(-3.356875,1.41314351751907E-16,0.846107820953206));
#13791=CARTESIAN_POINT('Ctrl Pts',(-3.33791387479986,0.0233367694770972,
0.844588565343252));
#13792=CARTESIAN_POINT('Ctrl Pts',(-3.31895541554339,0.0466702577927558,
0.842983206536337));
#13793=CARTESIAN_POINT('Ctrl Pts',(-3.3,0.07,0.841292647826788));
#13794=CARTESIAN_POINT('',(-3.356875,0.,1.5));
#13795=CARTESIAN_POINT('Origin',(-3.3,0.07,3.));
#13796=CARTESIAN_POINT('',(-3.243125,-5.25073838654019E-17,-0.0640355173918041));
#13797=CARTESIAN_POINT('Ctrl Pts',(-3.243125,0.,-0.0640355173918041));
#13798=CARTESIAN_POINT('Ctrl Pts',(-3.26208008208557,0.0233293317976187,
-0.062174805876581));
#13799=CARTESIAN_POINT('Ctrl Pts',(-3.28103854134525,0.0466628201172248,
-0.0603984498443344));
#13800=CARTESIAN_POINT('Ctrl Pts',(-3.3,0.07,-0.058707352173212));
#13801=CARTESIAN_POINT('',(-3.243125,5.3060421235922E-17,0.835964482608196));
#13802=CARTESIAN_POINT('',(-3.243125,0.,1.5));
#13803=CARTESIAN_POINT('Ctrl Pts',(-3.3,0.07,0.841292647826788));
#13804=CARTESIAN_POINT('Ctrl Pts',(-3.28103854134547,0.0466628201174959,
0.839601550155683));
#13805=CARTESIAN_POINT('Ctrl Pts',(-3.26208008208537,0.0233293317973772,
0.8378251941234));
#13806=CARTESIAN_POINT('Ctrl Pts',(-3.243125,1.31821497034025E-16,0.835964482608196));
#13807=CARTESIAN_POINT('Origin',(-3.765,-0.01,3.));
#13808=CARTESIAN_POINT('',(-3.7,0.07,-0.0360013659711851));
#13809=CARTESIAN_POINT('',(-3.756875,-5.46951915264603E-17,-0.0349329077078822));
#13810=CARTESIAN_POINT('Ctrl Pts',(-3.7,0.07,-0.0360013659711851));
#13811=CARTESIAN_POINT('Ctrl Pts',(-3.71895759470813,0.0466675757438436,
-0.0355535843916201));
#13812=CARTESIAN_POINT('Ctrl Pts',(-3.73791605423931,0.0233340870900765,
-0.0351971271763667));
#13813=CARTESIAN_POINT('Ctrl Pts',(-3.756875,0.,-0.0349329077078822));
#13814=CARTESIAN_POINT('',(-3.7,0.07,0.863998634028815));
#13815=CARTESIAN_POINT('',(-3.7,0.07,3.));
#13816=CARTESIAN_POINT('',(-3.756875,2.99479487072287E-16,0.865067092292118));
#13817=CARTESIAN_POINT('Ctrl Pts',(-3.756875,1.70945786985105E-16,0.865067092292118));
#13818=CARTESIAN_POINT('Ctrl Pts',(-3.73791605423931,0.0233340870900778,
0.864802872823633));
#13819=CARTESIAN_POINT('Ctrl Pts',(-3.71895759470813,0.0466675757438458,
0.86444641560838));
#13820=CARTESIAN_POINT('Ctrl Pts',(-3.7,0.07,0.863998634028815));
#13821=CARTESIAN_POINT('',(-3.756875,0.,1.5));
#13822=CARTESIAN_POINT('Origin',(-3.7,0.07,3.));
#13823=CARTESIAN_POINT('',(-3.643125,2.60349111665952E-16,-0.0376179427482956));
#13824=CARTESIAN_POINT('Ctrl Pts',(-3.643125,0.,-0.0376179427482956));
#13825=CARTESIAN_POINT('Ctrl Pts',(-3.66208223244517,0.0233319783940501,
-0.0369883513292489));
#13826=CARTESIAN_POINT('Ctrl Pts',(-3.68104069202526,0.0466654671080116,
-0.0364491880187094));
#13827=CARTESIAN_POINT('Ctrl Pts',(-3.7,0.07,-0.0360013659711851));
#13828=CARTESIAN_POINT('',(-3.643125,2.8345617330766E-16,0.862382057251704));
#13829=CARTESIAN_POINT('',(-3.643125,0.,1.5));
#13830=CARTESIAN_POINT('Ctrl Pts',(-3.7,0.07,0.863998634028815));
#13831=CARTESIAN_POINT('Ctrl Pts',(-3.68104069202525,0.0466654671079987,
0.86355081198129));
#13832=CARTESIAN_POINT('Ctrl Pts',(-3.66208223244515,0.0233319783940324,
0.863011648670751));
#13833=CARTESIAN_POINT('Ctrl Pts',(-3.643125,1.63126751949447E-16,0.862382057251704));
#13834=CARTESIAN_POINT('Origin',(-4.165,-0.01,3.));
#13835=CARTESIAN_POINT('',(-4.1,0.07,-0.0404236949732266));
#13836=CARTESIAN_POINT('',(-4.156875,1.35644074985623E-16,-0.0433654828435956));
#13837=CARTESIAN_POINT('Ctrl Pts',(-4.1,0.07,-0.0404236949732266));
#13838=CARTESIAN_POINT('Ctrl Pts',(-4.1189602801784,0.0466642705496571,
-0.0413061449568091));
#13839=CARTESIAN_POINT('Ctrl Pts',(-4.13791873829698,0.023330783634488,
-0.0422864363710023));
#13840=CARTESIAN_POINT('Ctrl Pts',(-4.156875,0.,-0.0433654828435955));
#13841=CARTESIAN_POINT('',(-4.1,0.07,0.859576305026773));
#13842=CARTESIAN_POINT('',(-4.1,0.07,3.));
#13843=CARTESIAN_POINT('',(-4.156875,2.91513808894911E-16,0.856634517156404));
#13844=CARTESIAN_POINT('Ctrl Pts',(-4.156875,1.94429843935443E-16,0.856634517156404));
#13845=CARTESIAN_POINT('Ctrl Pts',(-4.13791873829698,0.02333078363449,0.857713563628998));
#13846=CARTESIAN_POINT('Ctrl Pts',(-4.1189602801784,0.0466642705496608,
0.858693855043191));
#13847=CARTESIAN_POINT('Ctrl Pts',(-4.1,0.07,0.859576305026773));
#13848=CARTESIAN_POINT('',(-4.156875,0.,1.5));
#13849=CARTESIAN_POINT('Origin',(-4.1,0.07,3.));
#13850=CARTESIAN_POINT('',(-4.043125,-5.25073838654019E-17,-0.0380693521402107));
#13851=CARTESIAN_POINT('Ctrl Pts',(-4.043125,0.,-0.0380693521402107));
#13852=CARTESIAN_POINT('Ctrl Pts',(-4.06208488523803,0.0233352433698829,
-0.0387569372610109));
#13853=CARTESIAN_POINT('Ctrl Pts',(-4.08104334346688,0.0466687304207752,
-0.039541413641761));
#13854=CARTESIAN_POINT('Ctrl Pts',(-4.1,0.07,-0.0404236949732266));
#13855=CARTESIAN_POINT('',(-4.043125,9.65140495168372E-17,0.861930647859789));
#13856=CARTESIAN_POINT('',(-4.043125,0.,1.5));
#13857=CARTESIAN_POINT('Ctrl Pts',(-4.1,0.07,0.859576305026773));
#13858=CARTESIAN_POINT('Ctrl Pts',(-4.08104334346688,0.0466687304207743,
0.860458586358239));
#13859=CARTESIAN_POINT('Ctrl Pts',(-4.06208488523803,0.0233352433698813,
0.861243062738989));
#13860=CARTESIAN_POINT('Ctrl Pts',(-4.043125,1.88401971281291E-16,0.861930647859789));
#13861=CARTESIAN_POINT('Origin',(-4.565,-0.01,3.));
#13862=CARTESIAN_POINT('',(-4.5,0.07,-0.0739225060550655));
#13863=CARTESIAN_POINT('',(-4.556875,1.62444718833587E-16,-0.0811704877759833));
#13864=CARTESIAN_POINT('Ctrl Pts',(-4.5,0.07,-0.0739225060550655));
#13865=CARTESIAN_POINT('Ctrl Pts',(-4.51896356242444,0.0466602308622324,
-0.0762334807651054));
#13866=CARTESIAN_POINT('Ctrl Pts',(-4.53792201699023,0.0233267483197209,
-0.0786491744606242));
#13867=CARTESIAN_POINT('Ctrl Pts',(-4.556875,0.,-0.0811704877759835));
#13868=CARTESIAN_POINT('',(-4.5,0.07,0.826077493944934));
#13869=CARTESIAN_POINT('',(-4.5,0.07,3.));
#13870=CARTESIAN_POINT('',(-4.556875,1.14785019812011E-16,0.818829512224017));
#13871=CARTESIAN_POINT('Ctrl Pts',(-4.556875,2.11322032856213E-16,0.818829512224017));
#13872=CARTESIAN_POINT('Ctrl Pts',(-4.53792201699044,0.0233267483194611,
0.821350825539348));
#13873=CARTESIAN_POINT('Ctrl Pts',(-4.51896356242423,0.0466602308624903,
0.823766519234918));
#13874=CARTESIAN_POINT('Ctrl Pts',(-4.5,0.07,0.826077493944934));
#13875=CARTESIAN_POINT('',(-4.556875,0.,1.5));
#13876=CARTESIAN_POINT('Origin',(-4.5,0.07,3.));
#13877=CARTESIAN_POINT('',(-4.443125,-5.25073838654019E-17,-0.0673062343375367));
#13878=CARTESIAN_POINT('Ctrl Pts',(-4.443125,0.,-0.0673062343375367));
#13879=CARTESIAN_POINT('Ctrl Pts',(-4.4620881300192,0.0233392369467022,
-0.0694076443990267));
#13880=CARTESIAN_POINT('Ctrl Pts',(-4.48104658477782,0.0466727197265443,
-0.0716127679234912));
#13881=CARTESIAN_POINT('Ctrl Pts',(-4.5,0.07,-0.0739225060550655));
#13882=CARTESIAN_POINT('',(-4.443125,5.46327237080495E-16,0.832693765662463));
#13883=CARTESIAN_POINT('',(-4.443125,0.,1.5));
#13884=CARTESIAN_POINT('Ctrl Pts',(-4.5,0.07,0.826077493944934));
#13885=CARTESIAN_POINT('Ctrl Pts',(-4.48104658477761,0.0466727197262921,
0.828387232076536));
#13886=CARTESIAN_POINT('Ctrl Pts',(-4.46208813001941,0.0233392369469705,
0.830592355600949));
#13887=CARTESIAN_POINT('Ctrl Pts',(-4.443125,2.07217049616441E-16,0.832693765662464));
#13888=CARTESIAN_POINT('Origin',(-4.965,-0.01,3.));
#13889=CARTESIAN_POINT('',(-4.9,0.07,-0.13869094102463));
#13890=CARTESIAN_POINT('',(-4.956875,1.62444718833587E-16,-0.150579352803062));
#13891=CARTESIAN_POINT('Ctrl Pts',(-4.9,0.07,-0.13869094102463));
#13892=CARTESIAN_POINT('Ctrl Pts',(-4.91896754106353,0.0466553340756551,
-0.142541554477116));
#13893=CARTESIAN_POINT('Ctrl Pts',(-4.93792598942479,0.0233218591694844,
-0.146504068371518));
#13894=CARTESIAN_POINT('Ctrl Pts',(-4.956875,0.,-0.150579352803062));
#13895=CARTESIAN_POINT('',(-4.9,0.07,0.76130905897537));
#13896=CARTESIAN_POINT('',(-4.9,0.07,3.));
#13897=CARTESIAN_POINT('',(-4.956875,3.39810133618118E-16,0.749420647196938));
#13898=CARTESIAN_POINT('Ctrl Pts',(-4.956875,2.211215680057E-16,0.749420647196938));
#13899=CARTESIAN_POINT('Ctrl Pts',(-4.93792598942479,0.0233218591694845,
0.753495931628482));
#13900=CARTESIAN_POINT('Ctrl Pts',(-4.91896754106353,0.0466553340756546,
0.757458445522883));
#13901=CARTESIAN_POINT('Ctrl Pts',(-4.9,0.07,0.76130905897537));
#13902=CARTESIAN_POINT('',(-4.956875,1.11022302462516E-16,1.5));
#13903=CARTESIAN_POINT('Origin',(-4.9,0.07,3.));
#13904=CARTESIAN_POINT('',(-4.843125,1.33456267324564E-16,-0.127484356682433));
#13905=CARTESIAN_POINT('Ctrl Pts',(-4.843125,0.,-0.127484356682434));
#13906=CARTESIAN_POINT('Ctrl Pts',(-4.86209206517278,0.0233440802126523,
-0.131108755225662));
#13907=CARTESIAN_POINT('Ctrl Pts',(-4.88105051383643,0.0466775554909937,
-0.134843992909931));
#13908=CARTESIAN_POINT('Ctrl Pts',(-4.9,0.07,-0.13869094102463));
#13909=CARTESIAN_POINT('',(-4.843125,3.08788295873625E-16,0.772515643317567));
#13910=CARTESIAN_POINT('',(-4.843125,0.,1.5));
#13911=CARTESIAN_POINT('Ctrl Pts',(-4.9,0.07,0.76130905897537));
#13912=CARTESIAN_POINT('Ctrl Pts',(-4.88105051383644,0.0466775554909998,
0.765156007090068));
#13913=CARTESIAN_POINT('Ctrl Pts',(-4.86209206517279,0.0233440802126603,
0.768891244774337));
#13914=CARTESIAN_POINT('Ctrl Pts',(-4.843125,2.19088181770229E-16,0.772515643317567));
#13915=CARTESIAN_POINT('Origin',(-7.965,-0.01,3.));
#13916=CARTESIAN_POINT('',(-7.9,0.07,-1.94517408465831));
#13917=CARTESIAN_POINT('',(-7.956875,-8.17693113320588E-17,-2.0092495949436));
#13918=CARTESIAN_POINT('Ctrl Pts',(-7.9,0.07,-1.94517408465831));
#13919=CARTESIAN_POINT('Ctrl Pts',(-7.91903004493541,0.0465784062333396,
-1.96637153337838));
#13920=CARTESIAN_POINT('Ctrl Pts',(-7.93798830030226,0.0232451688587584,
-1.98773029266434));
#13921=CARTESIAN_POINT('Ctrl Pts',(-7.956875,0.,-2.0092495949436));
#13922=CARTESIAN_POINT('',(-7.9,0.07,-1.04517408465831));
#13923=CARTESIAN_POINT('',(-7.9,0.07,3.));
#13924=CARTESIAN_POINT('',(-7.956875,-8.63594602292614E-17,-1.1092495949436));
#13925=CARTESIAN_POINT('Ctrl Pts',(-7.956875,-5.68405272773159E-18,-1.1092495949436));
#13926=CARTESIAN_POINT('Ctrl Pts',(-7.93798830030226,0.0232451688587559,
-1.08773029266435));
#13927=CARTESIAN_POINT('Ctrl Pts',(-7.91903004493541,0.0465784062333384,
-1.06637153337838));
#13928=CARTESIAN_POINT('Ctrl Pts',(-7.9,0.07,-1.04517408465831));
#13929=CARTESIAN_POINT('',(-7.956875,0.,1.5));
#13930=CARTESIAN_POINT('Origin',(-7.9,0.07,3.));
#13931=CARTESIAN_POINT('',(-7.843125,-1.09390383052922E-16,-1.8825354103821));
#13932=CARTESIAN_POINT('Ctrl Pts',(-7.843125,0.,-1.88253541038209));
#13933=CARTESIAN_POINT('Ctrl Pts',(-7.86215375613703,0.0234200075532678,
-1.90325507663133));
#13934=CARTESIAN_POINT('Ctrl Pts',(-7.88111201563501,0.0467532500123186,
-1.92413487632433));
#13935=CARTESIAN_POINT('Ctrl Pts',(-7.9,0.07,-1.94517408465831));
#13936=CARTESIAN_POINT('',(-7.843125,-9.60410327554619E-17,-0.982535410382095));
#13937=CARTESIAN_POINT('',(-7.843125,2.22044604925031E-16,1.5));
#13938=CARTESIAN_POINT('Ctrl Pts',(-7.9,0.07,-1.04517408465831));
#13939=CARTESIAN_POINT('Ctrl Pts',(-7.88111201563501,0.0467532500123254,
-1.02413487632433));
#13940=CARTESIAN_POINT('Ctrl Pts',(-7.86215375613703,0.0234200075532716,
-1.00325507663133));
#13941=CARTESIAN_POINT('Ctrl Pts',(-7.843125,1.55371579585194E-17,-0.982535410382092));
#13942=CARTESIAN_POINT('Origin',(-5.565,-0.01,3.));
#13943=CARTESIAN_POINT('',(-5.5,0.07,-0.3));
#13944=CARTESIAN_POINT('',(-5.556875,1.62444718833587E-16,-0.319577961886773));
#13945=CARTESIAN_POINT('Ctrl Pts',(-5.5,0.07,-0.3));
#13946=CARTESIAN_POINT('Ctrl Pts',(-5.51897504895611,0.0466460935924786,
-0.30640268379866));
#13947=CARTESIAN_POINT('Ctrl Pts',(-5.53793348179804,0.0233126377870329,
-0.31292841138691));
#13948=CARTESIAN_POINT('Ctrl Pts',(-5.556875,0.,-0.319577961886773));
#13949=CARTESIAN_POINT('',(-5.5,0.07,0.6));
#13950=CARTESIAN_POINT('',(-5.5,0.07,3.));
#13951=CARTESIAN_POINT('',(-5.556875,3.39674161660188E-16,0.580422038113227));
#13952=CARTESIAN_POINT('Ctrl Pts',(-5.556875,2.21259072005402E-16,0.580422038113227));
#13953=CARTESIAN_POINT('Ctrl Pts',(-5.53793348179804,0.0233126377870342,
0.587071588613091));
#13954=CARTESIAN_POINT('Ctrl Pts',(-5.51897504895611,0.0466460935924807,
0.593597316201341));
#13955=CARTESIAN_POINT('Ctrl Pts',(-5.5,0.07,0.6));
#13956=CARTESIAN_POINT('',(-5.556875,0.,1.5));
#13957=CARTESIAN_POINT('Origin',(-5.5,0.07,3.));
#13958=CARTESIAN_POINT('',(-5.443125,1.64085574579381E-16,-0.281192597394316));
#13959=CARTESIAN_POINT('Ctrl Pts',(-5.443125,0.,-0.281192597394316));
#13960=CARTESIAN_POINT('Ctrl Pts',(-5.46209949275831,0.023353221856383,
-0.287339569361398));
#13961=CARTESIAN_POINT('Ctrl Pts',(-5.48105792614205,0.0466866783286795,
-0.293608442872478));
#13962=CARTESIAN_POINT('Ctrl Pts',(-5.5,0.07,-0.3));
#13963=CARTESIAN_POINT('',(-5.443125,3.42986627473185E-16,0.618807402605684));
#13964=CARTESIAN_POINT('',(-5.443125,-1.11022302462516E-16,1.5));
#13965=CARTESIAN_POINT('Ctrl Pts',(-5.5,0.07,0.6));
#13966=CARTESIAN_POINT('Ctrl Pts',(-5.48105792614205,0.0466866783286767,
0.606391557127523));
#13967=CARTESIAN_POINT('Ctrl Pts',(-5.46209949275831,0.0233532218563793,
0.612660430638604));
#13968=CARTESIAN_POINT('Ctrl Pts',(-5.443125,2.22657206114972E-16,0.618807402605684));
#13969=CARTESIAN_POINT('Origin',(-5.965,-0.01,3.));
#13970=CARTESIAN_POINT('',(-5.9,0.07,-0.454586831832013));
#13971=CARTESIAN_POINT('',(-5.956875,1.62444718833587E-16,-0.479861157396718));
#13972=CARTESIAN_POINT('Ctrl Pts',(-5.9,0.07,-0.454586831832013));
#13973=CARTESIAN_POINT('Ctrl Pts',(-5.91898124102904,0.0466384725796485,
-0.462880850871812));
#13974=CARTESIAN_POINT('Ctrl Pts',(-5.93793965850301,0.0233050356886025,
-0.471305400130083));
#13975=CARTESIAN_POINT('Ctrl Pts',(-5.956875,0.,-0.479861157396717));
#13976=CARTESIAN_POINT('',(-5.9,0.07,0.445413168167987));
#13977=CARTESIAN_POINT('',(-5.9,0.07,3.));
#13978=CARTESIAN_POINT('',(-5.956875,3.3154063110265E-16,0.420138842603282));
#13979=CARTESIAN_POINT('Ctrl Pts',(-5.956875,2.10664257829173E-16,0.420138842603282));
#13980=CARTESIAN_POINT('Ctrl Pts',(-5.93793965850301,0.0233050356886012,
0.428694599869916));
#13981=CARTESIAN_POINT('Ctrl Pts',(-5.91898124102904,0.0466384725796455,
0.437119149128187));
#13982=CARTESIAN_POINT('Ctrl Pts',(-5.9,0.07,0.445413168167987));
#13983=CARTESIAN_POINT('',(-5.956875,0.,1.5));
#13984=CARTESIAN_POINT('Origin',(-5.9,0.07,3.));
#13985=CARTESIAN_POINT('',(-5.843125,-8.31366911202204E-17,-0.430153510866633));
#13986=CARTESIAN_POINT('Ctrl Pts',(-5.843125,0.,-0.430153510866633));
#13987=CARTESIAN_POINT('Ctrl Pts',(-5.86210561773403,0.0233607602880359,
-0.438168384220962));
#13988=CARTESIAN_POINT('Ctrl Pts',(-5.88106403598116,0.0466941981306615,
-0.446312596977333));
#13989=CARTESIAN_POINT('Ctrl Pts',(-5.9,0.07,-0.454586831832013));
#13990=CARTESIAN_POINT('',(-5.843125,9.20861508289582E-17,0.469846489133368));
#13991=CARTESIAN_POINT('',(-5.843125,-1.11022302462516E-16,1.5));
#13992=CARTESIAN_POINT('Ctrl Pts',(-5.9,0.07,0.445413168167987));
#13993=CARTESIAN_POINT('Ctrl Pts',(-5.88106403598116,0.0466941981306552,
0.453687403022669));
#13994=CARTESIAN_POINT('Ctrl Pts',(-5.86210561773402,0.0233607602880265,
0.461831615779041));
#13995=CARTESIAN_POINT('Ctrl Pts',(-5.843125,2.1460337984823E-16,0.469846489133367));
#13996=CARTESIAN_POINT('Origin',(-6.365,-0.01,3.));
#13997=CARTESIAN_POINT('',(-6.3,0.07,-0.650817979540783));
#13998=CARTESIAN_POINT('',(-6.356875,-2.9918269764974E-16,-0.682328629485448));
#13999=CARTESIAN_POINT('Ctrl Pts',(-6.3,0.07,-0.650817979540783));
#14000=CARTESIAN_POINT('Ctrl Pts',(-6.31898850667717,0.0466295302434762,
-0.661183488938817));
#14001=CARTESIAN_POINT('Ctrl Pts',(-6.33794690403906,0.0232961181057714,
-0.671686861240141));
#14002=CARTESIAN_POINT('Ctrl Pts',(-6.356875,0.,-0.682328629485447));
#14003=CARTESIAN_POINT('',(-6.3,0.07,0.249182020459217));
#14004=CARTESIAN_POINT('',(-6.3,0.07,3.));
#14005=CARTESIAN_POINT('',(-6.356875,-1.46320085652327E-16,0.217671370514552));
#14006=CARTESIAN_POINT('Ctrl Pts',(-6.356875,1.90602294150671E-16,0.217671370514553));
#14007=CARTESIAN_POINT('Ctrl Pts',(-6.33794690403906,0.0232961181057672,
0.228313138759856));
#14008=CARTESIAN_POINT('Ctrl Pts',(-6.31898850667718,0.0466295302434675,
0.238816511061179));
#14009=CARTESIAN_POINT('Ctrl Pts',(-6.3,0.07,0.249182020459217));
#14010=CARTESIAN_POINT('',(-6.356875,0.,1.5));
#14011=CARTESIAN_POINT('Origin',(-6.3,0.07,3.));
#14012=CARTESIAN_POINT('',(-6.243125,-5.25073838654019E-17,-0.620230207960902));
#14013=CARTESIAN_POINT('Ctrl Pts',(-6.243125,0.,-0.620230207960902));
#14014=CARTESIAN_POINT('Ctrl Pts',(-6.2621128016042,0.0233696019744017,
-0.630289319492248));
#14015=CARTESIAN_POINT('Ctrl Pts',(-6.28107120005426,0.0467030154513895,
-0.640485063052609));
#14016=CARTESIAN_POINT('Ctrl Pts',(-6.3,0.07,-0.650817979540783));
#14017=CARTESIAN_POINT('',(-6.243125,1.05434277408689E-16,0.279769792039098));
#14018=CARTESIAN_POINT('',(-6.243125,0.,1.5));
#14019=CARTESIAN_POINT('Ctrl Pts',(-6.3,0.07,0.249182020459217));
#14020=CARTESIAN_POINT('Ctrl Pts',(-6.28107120005426,0.0467030154513984,
0.259514936947387));
#14021=CARTESIAN_POINT('Ctrl Pts',(-6.26211280160421,0.0233696019744131,
0.269710680507747));
#14022=CARTESIAN_POINT('Ctrl Pts',(-6.243125,1.97322199173142E-16,0.279769792039098));
#14023=CARTESIAN_POINT('Origin',(-6.765,-0.01,3.));
#14024=CARTESIAN_POINT('',(-6.7,0.07,-0.892754288213176));
#14025=CARTESIAN_POINT('',(-6.756875,-8.17693113320588E-17,-0.931132300718511));
#14026=CARTESIAN_POINT('Ctrl Pts',(-6.7,0.07,-0.892754288213176));
#14027=CARTESIAN_POINT('Ctrl Pts',(-6.71899694214736,0.046619148126331,
-0.905402013896704));
#14028=CARTESIAN_POINT('Ctrl Pts',(-6.73795531401288,0.0232857673687631,
-0.918194573745779));
#14029=CARTESIAN_POINT('Ctrl Pts',(-6.756875,0.,-0.931132300718512));
#14030=CARTESIAN_POINT('',(-6.7,0.07,0.00724571178682343));
#14031=CARTESIAN_POINT('',(-6.7,0.07,3.));
#14032=CARTESIAN_POINT('',(-6.756875,4.66488689181092E-17,-0.031132300718511));
#14033=CARTESIAN_POINT('Ctrl Pts',(-6.756875,1.60141391335515E-16,-0.0311323007185113));
#14034=CARTESIAN_POINT('Ctrl Pts',(-6.73795531401288,0.0232857673687599,
-0.0181945737457809));
#14035=CARTESIAN_POINT('Ctrl Pts',(-6.71899694214736,0.0466191481263249,
-0.00540201389670744));
#14036=CARTESIAN_POINT('Ctrl Pts',(-6.7,0.07,0.00724571178682343));
#14037=CARTESIAN_POINT('',(-6.756875,0.,1.5));
#14038=CARTESIAN_POINT('Origin',(-6.7,0.07,3.));
#14039=CARTESIAN_POINT('',(-6.643125,1.33456267324564E-16,-0.855395231580901));
#14040=CARTESIAN_POINT('Ctrl Pts',(-6.643125,0.,-0.855395231580901));
#14041=CARTESIAN_POINT('Ctrl Pts',(-6.66212113620276,0.0233798599418543,
-0.86770455853376));
#14042=CARTESIAN_POINT('Ctrl Pts',(-6.68107950958883,0.0467132425708651,
-0.880157462331309));
#14043=CARTESIAN_POINT('Ctrl Pts',(-6.7,0.07,-0.892754288213176));
#14044=CARTESIAN_POINT('',(-6.643125,2.7056128390321E-16,0.0446047684190993));
#14045=CARTESIAN_POINT('',(-6.643125,0.,1.5));
#14046=CARTESIAN_POINT('Ctrl Pts',(-6.7,0.07,0.00724571178682343));
#14047=CARTESIAN_POINT('Ctrl Pts',(-6.68107950958883,0.0467132425708681,
0.0198425376686894));
#14048=CARTESIAN_POINT('Ctrl Pts',(-6.66212113620276,0.0233798599418581,
0.0322954414662376));
#14049=CARTESIAN_POINT('Ctrl Pts',(-6.643125,1.69922131494523E-16,0.0446047684190992));
#14050=CARTESIAN_POINT('Origin',(-7.165,-0.01,3.));
#14051=CARTESIAN_POINT('',(-7.1,0.07,-1.18516288868335));
#14052=CARTESIAN_POINT('',(-7.156875,5.4312325185776E-16,-1.23115344810839));
#14053=CARTESIAN_POINT('Ctrl Pts',(-7.1,0.07,-1.18516288868335));
#14054=CARTESIAN_POINT('Ctrl Pts',(-7.11900663042154,0.0466072240965719,
-1.20034183864505));
#14055=CARTESIAN_POINT('Ctrl Pts',(-7.13796497071894,0.0232738821920808,
-1.21567200422041));
#14056=CARTESIAN_POINT('Ctrl Pts',(-7.156875,0.,-1.23115344810839));
#14057=CARTESIAN_POINT('',(-7.1,0.07,-0.28516288868335));
#14058=CARTESIAN_POINT('',(-7.1,0.07,3.));
#14059=CARTESIAN_POINT('',(-7.156875,6.38063870818107E-16,-0.331153448108389));
#14060=CARTESIAN_POINT('Ctrl Pts',(-7.156875,1.18186075359093E-16,-0.33115344810839));
#14061=CARTESIAN_POINT('Ctrl Pts',(-7.13796497071891,0.0232738821921115,
-0.31567200422039));
#14062=CARTESIAN_POINT('Ctrl Pts',(-7.11900663042157,0.046607224096525,
-0.300341838645079));
#14063=CARTESIAN_POINT('Ctrl Pts',(-7.1,0.07,-0.28516288868335));
#14064=CARTESIAN_POINT('',(-7.156875,-2.22044604925031E-16,1.5));
#14065=CARTESIAN_POINT('Origin',(-7.1,0.07,3.));
#14066=CARTESIAN_POINT('',(-7.043125,1.33456267324564E-16,-1.14030527259989));
#14067=CARTESIAN_POINT('Ctrl Pts',(-7.043125,0.,-1.14030527259989));
#14068=CARTESIAN_POINT('Ctrl Pts',(-7.06213069882356,0.0233916293213094,
-1.15510783188482));
#14069=CARTESIAN_POINT('Ctrl Pts',(-7.08108904123993,0.0467249738337627,
-1.1700603433936));
#14070=CARTESIAN_POINT('Ctrl Pts',(-7.1,0.07,-1.18516288868335));
#14071=CARTESIAN_POINT('',(-7.043125,6.76122212833369E-16,-0.240305272599889));
#14072=CARTESIAN_POINT('',(-7.043125,0.,1.5));
#14073=CARTESIAN_POINT('Ctrl Pts',(-7.1,0.07,-0.28516288868335));
#14074=CARTESIAN_POINT('Ctrl Pts',(-7.08108904123999,0.0467249738338329,
-0.270060343393643));
#14075=CARTESIAN_POINT('Ctrl Pts',(-7.06213069882353,0.0233916293212594,
-0.255107831884786));
#14076=CARTESIAN_POINT('Ctrl Pts',(-7.043125,1.3135810522982E-16,-0.24030527259989));
#14077=CARTESIAN_POINT('Origin',(-7.565,-0.01,3.));
#14078=CARTESIAN_POINT('',(-7.5,0.07,-1.53370216351703));
#14079=CARTESIAN_POINT('',(-7.556875,-8.17693113320588E-17,-1.58819576970747));
#14080=CARTESIAN_POINT('Ctrl Pts',(-7.5,0.07,-1.53370216351703));
#14081=CARTESIAN_POINT('Ctrl Pts',(-7.51901764211564,0.0465936712422835,
-1.55171002089042));
#14082=CARTESIAN_POINT('Ctrl Pts',(-7.53797594395267,0.0232603766736332,
-1.5698746550546));
#14083=CARTESIAN_POINT('Ctrl Pts',(-7.556875,0.,-1.58819576970747));
#14084=CARTESIAN_POINT('',(-7.5,0.07,-0.633702163517027));
#14085=CARTESIAN_POINT('',(-7.5,0.07,3.));
#14086=CARTESIAN_POINT('',(-7.556875,-3.09153462868992E-17,-0.688195769707468));
#14087=CARTESIAN_POINT('Ctrl Pts',(-7.556875,6.34338590962456E-17,-0.688195769707468));
#14088=CARTESIAN_POINT('Ctrl Pts',(-7.53797594395267,0.0232603766736338,
-0.669874655054604));
#14089=CARTESIAN_POINT('Ctrl Pts',(-7.51901764211564,0.0465936712422837,
-0.651710020890421));
#14090=CARTESIAN_POINT('Ctrl Pts',(-7.5,0.07,-0.633702163517027));
#14091=CARTESIAN_POINT('',(-7.556875,0.,1.5));
#14092=CARTESIAN_POINT('Origin',(-7.5,0.07,3.));
#14093=CARTESIAN_POINT('',(-7.443125,-8.31366911202204E-17,-1.48047844752676));
#14094=CARTESIAN_POINT('Ctrl Pts',(-7.443125,0.,-1.48047844752676));
#14095=CARTESIAN_POINT('Ctrl Pts',(-7.46214155275804,0.0234049880098914,
-1.49806423898676));
#14096=CARTESIAN_POINT('Ctrl Pts',(-7.48109985754961,0.046738286214905,
-1.51580556689828));
#14097=CARTESIAN_POINT('Ctrl Pts',(-7.5,0.07,-1.53370216351703));
#14098=CARTESIAN_POINT('',(-7.443125,-1.80596202401722E-17,-0.580478447526757));
#14099=CARTESIAN_POINT('',(-7.443125,-2.22044604925031E-16,1.5));
#14100=CARTESIAN_POINT('Ctrl Pts',(-7.5,0.07,-0.633702163517027));
#14101=CARTESIAN_POINT('Ctrl Pts',(-7.48109985754962,0.0467382862149124,
-0.615805566898287));
#14102=CARTESIAN_POINT('Ctrl Pts',(-7.46214155275804,0.0234049880098951,
-0.598064238986766));
#14103=CARTESIAN_POINT('Ctrl Pts',(-7.443125,8.03917245074572E-17,-0.580478447526758));
#14104=CARTESIAN_POINT('Origin',(-7.765,-0.01,3.));
#14105=CARTESIAN_POINT('',(-7.7,0.07,-1.73109299233075));
#14106=CARTESIAN_POINT('',(-7.756875,-8.17693113320588E-17,-1.79022880539828));
#14107=CARTESIAN_POINT('Ctrl Pts',(-7.7,0.07,-1.73109299233075));
#14108=CARTESIAN_POINT('Ctrl Pts',(-7.71902366500654,0.0465862584534947,
-1.75064591874077));
#14109=CARTESIAN_POINT('Ctrl Pts',(-7.73798194469789,0.0232529911410549,
-1.77035802849347));
#14110=CARTESIAN_POINT('Ctrl Pts',(-7.756875,0.,-1.79022880539828));
#14111=CARTESIAN_POINT('',(-7.7,0.07,-0.83109299233075));
#14112=CARTESIAN_POINT('',(-7.7,0.07,3.));
#14113=CARTESIAN_POINT('',(-7.756875,-5.70046523168335E-17,-0.890228805398279));
#14114=CARTESIAN_POINT('Ctrl Pts',(-7.756875,3.07811300831359E-17,-0.89022880539828));
#14115=CARTESIAN_POINT('Ctrl Pts',(-7.73798194469789,0.0232529911410541,
-0.870358028493467));
#14116=CARTESIAN_POINT('Ctrl Pts',(-7.71902366500654,0.0465862584534942,
-0.850645918740776));
#14117=CARTESIAN_POINT('Ctrl Pts',(-7.7,0.07,-0.83109299233075));
#14118=CARTESIAN_POINT('',(-7.756875,0.,1.5));
#14119=CARTESIAN_POINT('Origin',(-7.7,0.07,3.));
#14120=CARTESIAN_POINT('',(-7.643125,-8.31366911202204E-17,-1.67330624992589));
#14121=CARTESIAN_POINT('Ctrl Pts',(-7.643125,0.,-1.67330624992589));
#14122=CARTESIAN_POINT('Ctrl Pts',(-7.66214748185074,0.0234122853547581,
-1.69241068899391));
#14123=CARTESIAN_POINT('Ctrl Pts',(-7.68110576503403,0.0467455569649661,
-1.71167309686182));
#14124=CARTESIAN_POINT('Ctrl Pts',(-7.7,0.07,-1.73109299233075));
#14125=CARTESIAN_POINT('',(-7.643125,-4.42708618374973E-17,-0.773306249925886));
#14126=CARTESIAN_POINT('',(-7.643125,2.22044604925031E-16,1.5));
#14127=CARTESIAN_POINT('Ctrl Pts',(-7.7,0.07,-0.83109299233075));
#14128=CARTESIAN_POINT('Ctrl Pts',(-7.68110576503403,0.0467455569649649,
-0.811673096861818));
#14129=CARTESIAN_POINT('Ctrl Pts',(-7.66214748185074,0.0234122853547573,
-0.792410688993914));
#14130=CARTESIAN_POINT('Ctrl Pts',(-7.643125,4.98048675880153E-17,-0.773306249925886));
#14131=CARTESIAN_POINT('Origin',(-7.365,-0.01,3.));
#14132=CARTESIAN_POINT('',(-7.3,0.07,-1.35202141064204));
#14133=CARTESIAN_POINT('',(-7.356875,-5.1632260800979E-16,-1.40214159053033));
#14134=CARTESIAN_POINT('Ctrl Pts',(-7.3,0.07,-1.35202141064204));
#14135=CARTESIAN_POINT('Ctrl Pts',(-7.31901196673093,0.0466006563311587,
-1.36857405949961));
#14136=CARTESIAN_POINT('Ctrl Pts',(-7.33797028871996,0.0232673369600475,
-1.3852808209203));
#14137=CARTESIAN_POINT('Ctrl Pts',(-7.356875,0.,-1.40214159053033));
#14138=CARTESIAN_POINT('',(-7.3,0.07,-0.452021410642036));
#14139=CARTESIAN_POINT('',(-7.3,0.07,3.));
#14140=CARTESIAN_POINT('',(-7.356875,-7.59164575381956E-18,-0.502141590530332));
#14141=CARTESIAN_POINT('Ctrl Pts',(-7.356875,9.25005547396034E-17,-0.502141590530333));
#14142=CARTESIAN_POINT('Ctrl Pts',(-7.33797028871987,0.0232673369601652,
-0.485280820920213));
#14143=CARTESIAN_POINT('Ctrl Pts',(-7.319011966731,0.0466006563310788,-0.468574059499668));
#14144=CARTESIAN_POINT('Ctrl Pts',(-7.3,0.07,-0.452021410642036));
#14145=CARTESIAN_POINT('',(-7.356875,0.,1.5));
#14146=CARTESIAN_POINT('Origin',(-7.3,0.07,3.));
#14147=CARTESIAN_POINT('',(-7.243125,-8.31366911202204E-17,-1.3030993940485));
#14148=CARTESIAN_POINT('Ctrl Pts',(-7.243125,0.,-1.3030993940485));
#14149=CARTESIAN_POINT('Ctrl Pts',(-7.26213596080226,0.0233981056027806,
-1.31925390353022));
#14150=CARTESIAN_POINT('Ctrl Pts',(-7.28109428529282,0.0467314280527045,
-1.33556126943843));
#14151=CARTESIAN_POINT('Ctrl Pts',(-7.3,0.07,-1.35202141064204));
#14152=CARTESIAN_POINT('',(-7.243125,2.49674900947315E-18,-0.4030993940485));
#14153=CARTESIAN_POINT('',(-7.243125,2.22044604925031E-16,1.5));
#14154=CARTESIAN_POINT('Ctrl Pts',(-7.3,0.07,-0.452021410642036));
#14155=CARTESIAN_POINT('Ctrl Pts',(-7.28109428529286,0.0467314280527458,
-0.435561269438458));
#14156=CARTESIAN_POINT('Ctrl Pts',(-7.2621359608022,0.0233981056027132,
-0.419253903530172));
#14157=CARTESIAN_POINT('Ctrl Pts',(-7.243125,1.07511516740278E-16,-0.403099394048499));
#14158=CARTESIAN_POINT('Origin',(-6.965,-0.01,3.));
#14159=CARTESIAN_POINT('',(-6.9,0.07,-1.03231935622351));
#14160=CARTESIAN_POINT('',(-6.956875,-2.9918269764974E-16,-1.07440225892494));
#14161=CARTESIAN_POINT('Ctrl Pts',(-6.9,0.07,-1.03231935622351));
#14162=CARTESIAN_POINT('Ctrl Pts',(-6.91900162503864,0.046613384567828,
-1.0461988079961));
#14163=CARTESIAN_POINT('Ctrl Pts',(-6.93795998192576,0.0232800222452229,
-1.0602263730092));
#14164=CARTESIAN_POINT('Ctrl Pts',(-6.956875,0.,-1.07440225892494));
#14165=CARTESIAN_POINT('',(-6.9,0.07,-0.132319356223514));
#14166=CARTESIAN_POINT('',(-6.9,0.07,3.));
#14167=CARTESIAN_POINT('',(-6.956875,-1.86400758421015E-16,-0.174402258924944));
#14168=CARTESIAN_POINT('Ctrl Pts',(-6.956875,1.4067648690722E-16,-0.174402258924944));
#14169=CARTESIAN_POINT('Ctrl Pts',(-6.93795998192544,0.0232800222456121,
-0.160226373008964));
#14170=CARTESIAN_POINT('Ctrl Pts',(-6.91900162503897,0.0466133845674241,
-0.146198807996338));
#14171=CARTESIAN_POINT('Ctrl Pts',(-6.9,0.07,-0.132319356223514));
#14172=CARTESIAN_POINT('',(-6.956875,0.,1.5));
#14173=CARTESIAN_POINT('Origin',(-6.9,0.07,3.));
#14174=CARTESIAN_POINT('',(-6.843125,-1.09390383052922E-16,-0.991309886408041));
#14175=CARTESIAN_POINT('Ctrl Pts',(-6.843125,0.,-0.991309886408041));
#14176=CARTESIAN_POINT('Ctrl Pts',(-6.86212575977902,0.0233855504972543,
-1.00483278553493));
#14177=CARTESIAN_POINT('Ctrl Pts',(-6.88108411846137,0.046718915029381,
-1.0185025345034));
#14178=CARTESIAN_POINT('Ctrl Pts',(-6.9,0.07,-1.03231935622351));
#14179=CARTESIAN_POINT('',(-6.843125,1.20882408210842E-17,-0.0913098864080408));
#14180=CARTESIAN_POINT('',(-6.843125,0.,1.5));
#14181=CARTESIAN_POINT('Ctrl Pts',(-6.9,0.07,-0.132319356223514));
#14182=CARTESIAN_POINT('Ctrl Pts',(-6.88108411846138,0.0467189150293865,
-0.118502534503401));
#14183=CARTESIAN_POINT('Ctrl Pts',(-6.86212575977903,0.0233855504972626,
-0.104832785534938));
#14184=CARTESIAN_POINT('Ctrl Pts',(-6.843125,1.52107931128825E-16,-0.0913098864080409));
#14185=CARTESIAN_POINT('Origin',(-6.565,-0.01,3.));
#14186=CARTESIAN_POINT('',(-6.5,0.07,-0.765793495486731));
#14187=CARTESIAN_POINT('',(-6.556875,-8.17693113320588E-17,-0.800652433967885));
#14188=CARTESIAN_POINT('Ctrl Pts',(-6.5,0.07,-0.765793495486731));
#14189=CARTESIAN_POINT('Ctrl Pts',(-6.51899257266672,0.0466245259486468,
-0.777271587041565));
#14190=CARTESIAN_POINT('Ctrl Pts',(-6.53795095799464,0.0232911286219822,
-0.788891086279516));
#14191=CARTESIAN_POINT('Ctrl Pts',(-6.556875,0.,-0.800652433967885));
#14192=CARTESIAN_POINT('',(-6.5,0.07,0.134206504513269));
#14193=CARTESIAN_POINT('',(-6.5,0.07,3.));
#14194=CARTESIAN_POINT('',(-6.556875,5.99616627919403E-17,0.0993475660321151));
#14195=CARTESIAN_POINT('Ctrl Pts',(-6.556875,1.76735896700934E-16,0.0993475660321151));
#14196=CARTESIAN_POINT('Ctrl Pts',(-6.53795095799464,0.0232911286219812,
0.111108913720483));
#14197=CARTESIAN_POINT('Ctrl Pts',(-6.51899257266672,0.0466245259486444,
0.122728412958434));
#14198=CARTESIAN_POINT('Ctrl Pts',(-6.5,0.07,0.134206504513269));
#14199=CARTESIAN_POINT('',(-6.556875,0.,1.5));
#14200=CARTESIAN_POINT('Origin',(-6.5,0.07,3.));
#14201=CARTESIAN_POINT('',(-6.443125,1.33456267324564E-16,-0.731903492805105));
#14202=CARTESIAN_POINT('Ctrl Pts',(-6.443125,0.,-0.731903492805105));
#14203=CARTESIAN_POINT('Ctrl Pts',(-6.46211681986679,0.0233745475283574,
-0.743059848656298));
#14204=CARTESIAN_POINT('Ctrl Pts',(-6.48107520648177,0.046707946439098,
-0.754356366011439));
#14205=CARTESIAN_POINT('Ctrl Pts',(-6.5,0.07,-0.765793495486731));
#14206=CARTESIAN_POINT('',(-6.443125,2.83399680390998E-16,0.168096507194895));
#14207=CARTESIAN_POINT('',(-6.443125,0.,1.5));
#14208=CARTESIAN_POINT('Ctrl Pts',(-6.5,0.07,0.134206504513269));
#14209=CARTESIAN_POINT('Ctrl Pts',(-6.48107520648177,0.0467079464391011,
0.14564363398856));
#14210=CARTESIAN_POINT('Ctrl Pts',(-6.46211681986679,0.0233745475283613,
0.1569401513437));
#14211=CARTESIAN_POINT('Ctrl Pts',(-6.443125,1.84948335643369E-16,0.168096507194895));
#14212=CARTESIAN_POINT('Origin',(-6.165,-0.01,3.));
#14213=CARTESIAN_POINT('',(-6.1,0.07,-0.547257807070654));
#14214=CARTESIAN_POINT('',(-6.156875,-2.9918269764974E-16,-0.575577572177906));
#14215=CARTESIAN_POINT('Ctrl Pts',(-6.1,0.07,-0.547257807070654));
#14216=CARTESIAN_POINT('Ctrl Pts',(-6.11898473335907,0.0466341743272997,
-0.556563296824527));
#14217=CARTESIAN_POINT('Ctrl Pts',(-6.13794314140949,0.0233007490344763,
-0.56600301468492));
#14218=CARTESIAN_POINT('Ctrl Pts',(-6.156875,0.,-0.575577572177906));
#14219=CARTESIAN_POINT('',(-6.1,0.07,0.352742192929346));
#14220=CARTESIAN_POINT('',(-6.1,0.07,3.));
#14221=CARTESIAN_POINT('',(-6.156875,5.15001464878538E-16,0.324422427822094));
#14222=CARTESIAN_POINT('Ctrl Pts',(-6.156875,2.0187149338955E-16,0.324422427822093));
#14223=CARTESIAN_POINT('Ctrl Pts',(-6.13794314140949,0.0233007490344754,
0.333996985315079));
#14224=CARTESIAN_POINT('Ctrl Pts',(-6.11898473335907,0.0466341743272964,
0.343436703175472));
#14225=CARTESIAN_POINT('Ctrl Pts',(-6.1,0.07,0.352742192929346));
#14226=CARTESIAN_POINT('',(-6.156875,0.,1.5));
#14227=CARTESIAN_POINT('Origin',(-6.1,0.07,3.));
#14228=CARTESIAN_POINT('',(-6.043125,-5.25073838654019E-17,-0.519818399548886));
#14229=CARTESIAN_POINT('Ctrl Pts',(-6.043125,0.,-0.519818399548886));
#14230=CARTESIAN_POINT('Ctrl Pts',(-6.06210907125938,0.0233650107807755,
-0.528831646889548));
#14231=CARTESIAN_POINT('Ctrl Pts',(-6.08106748022819,0.0466984372039219,
-0.537977910144092));
#14232=CARTESIAN_POINT('Ctrl Pts',(-6.1,0.07,-0.547257807070654));
#14233=CARTESIAN_POINT('',(-6.043125,5.46278908473655E-16,0.380181600451114));
#14234=CARTESIAN_POINT('',(-6.043125,1.11022302462516E-16,1.5));
#14235=CARTESIAN_POINT('Ctrl Pts',(-6.1,0.07,0.352742192929346));
#14236=CARTESIAN_POINT('Ctrl Pts',(-6.08106748022819,0.0466984372039235,
0.362022089855907));
#14237=CARTESIAN_POINT('Ctrl Pts',(-6.06210907125938,0.0233650107807784,
0.371168353110451));
#14238=CARTESIAN_POINT('Ctrl Pts',(-6.043125,2.07168721009601E-16,0.380181600451114));
#14239=CARTESIAN_POINT('Origin',(-5.765,-0.01,3.));
#14240=CARTESIAN_POINT('',(-5.7,0.07,-0.372318124828976));
#14241=CARTESIAN_POINT('',(-5.756875,-5.46951915264603E-17,-0.394681732200484));
#14242=CARTESIAN_POINT('Ctrl Pts',(-5.7,0.07,-0.372318124828976));
#14243=CARTESIAN_POINT('Ctrl Pts',(-5.71897801724519,0.0466424403136126,
-0.379645621801429));
#14244=CARTESIAN_POINT('Ctrl Pts',(-5.73793644295687,0.0233089932838593,
-0.387099913179927));
#14245=CARTESIAN_POINT('Ctrl Pts',(-5.756875,0.,-0.394681732200484));
#14246=CARTESIAN_POINT('',(-5.7,0.07,0.527681875171024));
#14247=CARTESIAN_POINT('',(-5.7,0.07,3.));
#14248=CARTESIAN_POINT('',(-5.756875,1.19461355686473E-16,0.505318267799516));
#14249=CARTESIAN_POINT('Ctrl Pts',(-5.756875,2.17092272561204E-16,0.505318267799516));
#14250=CARTESIAN_POINT('Ctrl Pts',(-5.73793644295687,0.0233089932838589,
0.512900086820073));
#14251=CARTESIAN_POINT('Ctrl Pts',(-5.71897801724519,0.0466424403136115,
0.52035437819857));
#14252=CARTESIAN_POINT('Ctrl Pts',(-5.7,0.07,0.527681875171024));
#14253=CARTESIAN_POINT('',(-5.756875,-1.11022302462516E-16,1.5));
#14254=CARTESIAN_POINT('Origin',(-5.7,0.07,3.));
#14255=CARTESIAN_POINT('',(-5.643125,1.33456267324564E-16,-0.350759016032021));
#14256=CARTESIAN_POINT('Ctrl Pts',(-5.643125,0.,-0.350759016032021));
#14257=CARTESIAN_POINT('Ctrl Pts',(-5.66210242910056,0.023356835816077,
-0.357819512870387));
#14258=CARTESIAN_POINT('Ctrl Pts',(-5.68106085546093,0.0466902836442217,
-0.365005636781582));
#14259=CARTESIAN_POINT('Ctrl Pts',(-5.7,0.07,-0.372318124828976));
#14260=CARTESIAN_POINT('',(-5.643125,3.09433233472242E-16,0.549240983967979));
#14261=CARTESIAN_POINT('',(-5.643125,0.,1.5));
#14262=CARTESIAN_POINT('Ctrl Pts',(-5.7,0.07,0.527681875171024));
#14263=CARTESIAN_POINT('Ctrl Pts',(-5.68106085546092,0.0466902836442103,
0.534994363218421));
#14264=CARTESIAN_POINT('Ctrl Pts',(-5.66210242910055,0.023356835816061,
0.542180487129618));
#14265=CARTESIAN_POINT('Ctrl Pts',(-5.643125,2.19733119368846E-16,0.549240983967978));
#14266=CARTESIAN_POINT('Origin',(-5.365,-0.01,3.));
#14267=CARTESIAN_POINT('',(-5.3,0.07,-0.237212543217153));
#14268=CARTESIAN_POINT('',(-5.356875,3.53057461303304E-16,-0.25412122421867));
#14269=CARTESIAN_POINT('Ctrl Pts',(-5.3,0.07,-0.237212543217153));
#14270=CARTESIAN_POINT('Ctrl Pts',(-5.31897232267343,0.0466494490173111,
-0.242729198765226));
#14271=CARTESIAN_POINT('Ctrl Pts',(-5.33793076161593,0.0233159857034724,
-0.248365153574487));
#14272=CARTESIAN_POINT('Ctrl Pts',(-5.356875,0.,-0.25412122421867));
#14273=CARTESIAN_POINT('',(-5.3,0.07,0.662787456782847));
#14274=CARTESIAN_POINT('',(-5.3,0.07,3.));
#14275=CARTESIAN_POINT('',(-5.356875,5.32015205297343E-16,0.64587877578133));
#14276=CARTESIAN_POINT('Ctrl Pts',(-5.356875,2.23260849130472E-16,0.64587877578133));
#14277=CARTESIAN_POINT('Ctrl Pts',(-5.33793076161593,0.0233159857034787,
0.651634846425515));
#14278=CARTESIAN_POINT('Ctrl Pts',(-5.31897232267342,0.0466494490173225,
0.657270801234777));
#14279=CARTESIAN_POINT('Ctrl Pts',(-5.3,0.07,0.662787456782847));
#14280=CARTESIAN_POINT('',(-5.356875,0.,1.5));
#14281=CARTESIAN_POINT('Origin',(-5.3,0.07,3.));
#14282=CARTESIAN_POINT('',(-5.243125,1.64085574579381E-16,-0.221042803198048));
#14283=CARTESIAN_POINT('Ctrl Pts',(-5.243125,0.,-0.221042803198049));
#14284=CARTESIAN_POINT('Ctrl Pts',(-5.26209679561258,0.0233499022924093,
-0.226314260319612));
#14285=CARTESIAN_POINT('Ctrl Pts',(-5.28105523500498,0.0466833661599716,
-0.231703900721854));
#14286=CARTESIAN_POINT('Ctrl Pts',(-5.3,0.07,-0.237212543217153));
#14287=CARTESIAN_POINT('',(-5.243125,5.60390359396119E-16,0.678957196801951));
#14288=CARTESIAN_POINT('',(-5.243125,0.,1.5));
#14289=CARTESIAN_POINT('Ctrl Pts',(-5.3,0.07,0.662787456782847));
#14290=CARTESIAN_POINT('Ctrl Pts',(-5.28105523500499,0.0466833661599827,
0.668296099278144));
#14291=CARTESIAN_POINT('Ctrl Pts',(-5.2620967956126,0.0233499022924248,
0.673685739680385));
#14292=CARTESIAN_POINT('Ctrl Pts',(-5.243125,2.23467979593124E-16,0.678957196801951));
#14293=CARTESIAN_POINT('Origin',(-5.165,-0.01,3.));
#14294=CARTESIAN_POINT('',(-5.1,0.07,-0.183564568819186));
#14295=CARTESIAN_POINT('',(-5.156875,-8.17693113320588E-17,-0.197912451271776));
#14296=CARTESIAN_POINT('Ctrl Pts',(-5.1,0.07,-0.183564568819186));
#14297=CARTESIAN_POINT('Ctrl Pts',(-5.11896982465166,0.0466525235056449,
-0.188231334707976));
#14298=CARTESIAN_POINT('Ctrl Pts',(-5.13792826874203,0.0233190538559675,
-0.193013679992787));
#14299=CARTESIAN_POINT('Ctrl Pts',(-5.156875,0.,-0.197912451271776));
#14300=CARTESIAN_POINT('',(-5.1,0.07,0.716435431180814));
#14301=CARTESIAN_POINT('',(-5.1,0.07,3.));
#14302=CARTESIAN_POINT('',(-5.156875,3.14528134067499E-16,0.702087548728224));
#14303=CARTESIAN_POINT('Ctrl Pts',(-5.156875,2.23187164218309E-16,0.702087548728225));
#14304=CARTESIAN_POINT('Ctrl Pts',(-5.13792826874202,0.0233190538559761,
0.706986320007216));
#14305=CARTESIAN_POINT('Ctrl Pts',(-5.11896982465165,0.0466525235056635,
0.711768665292028));
#14306=CARTESIAN_POINT('Ctrl Pts',(-5.1,0.07,0.716435431180814));
#14307=CARTESIAN_POINT('',(-5.156875,0.,1.5));
#14308=CARTESIAN_POINT('Origin',(-5.1,0.07,3.));
#14309=CARTESIAN_POINT('',(-5.043125,-2.71288149971243E-16,-0.169926113751101));
#14310=CARTESIAN_POINT('Ctrl Pts',(-5.043125,0.,-0.169926113751102));
#14311=CARTESIAN_POINT('Ctrl Pts',(-5.06209432426069,0.023346860628547,
-0.174357492189475));
#14312=CARTESIAN_POINT('Ctrl Pts',(-5.08105276872176,0.0466803307344779,
-0.178903361125593));
#14313=CARTESIAN_POINT('Ctrl Pts',(-5.1,0.07,-0.183564568819186));
#14314=CARTESIAN_POINT('',(-5.043125,1.25987973607517E-16,0.730073886248899));
#14315=CARTESIAN_POINT('',(-5.043125,1.11022302462516E-16,1.5));
#14316=CARTESIAN_POINT('Ctrl Pts',(-5.1,0.07,0.716435431180814));
#14317=CARTESIAN_POINT('Ctrl Pts',(-5.08105276872176,0.0466803307344801,
0.721096638874407));
#14318=CARTESIAN_POINT('Ctrl Pts',(-5.0620943242607,0.0233468606285505,
0.725642507810524));
#14319=CARTESIAN_POINT('Ctrl Pts',(-5.043125,2.22251510694087E-16,0.730073886248899));
#14320=CARTESIAN_POINT('Origin',(-4.765,-0.01,3.));
#14321=CARTESIAN_POINT('',(-4.7,0.07,-0.102250208141538));
#14322=CARTESIAN_POINT('',(-4.756875,1.62444718833587E-16,-0.11177396627754));
#14323=CARTESIAN_POINT('Ctrl Pts',(-4.7,0.07,-0.102250208141538));
#14324=CARTESIAN_POINT('Ctrl Pts',(-4.71896545816211,0.0466578976466294,
-0.105316221858779));
#14325=CARTESIAN_POINT('Ctrl Pts',(-4.7379239099913,0.0233244184722453,
-0.108490511947973));
#14326=CARTESIAN_POINT('Ctrl Pts',(-4.756875,0.,-0.11177396627754));
#14327=CARTESIAN_POINT('',(-4.7,0.07,0.797749791858462));
#14328=CARTESIAN_POINT('',(-4.7,0.07,3.));
#14329=CARTESIAN_POINT('',(-4.756875,1.1951123464156E-16,0.78822603372246));
#14330=CARTESIAN_POINT('Ctrl Pts',(-4.756875,2.17142151516292E-16,0.78822603372246));
#14331=CARTESIAN_POINT('Ctrl Pts',(-4.73792390999119,0.0233244184723788,
0.791509488052046));
#14332=CARTESIAN_POINT('Ctrl Pts',(-4.71896545816221,0.0466578976465091,
0.794683778141207));
#14333=CARTESIAN_POINT('Ctrl Pts',(-4.7,0.07,0.797749791858462));
#14334=CARTESIAN_POINT('',(-4.756875,0.,1.5));
#14335=CARTESIAN_POINT('Origin',(-4.7,0.07,3.));
#14336=CARTESIAN_POINT('',(-4.643125,-8.31366911202204E-17,-0.0933824218252977));
#14337=CARTESIAN_POINT('Ctrl Pts',(-4.643125,0.,-0.0933824218252975));
#14338=CARTESIAN_POINT('Ctrl Pts',(-4.6620900048594,0.0233415444423344,
-0.0962308114370454));
#14339=CARTESIAN_POINT('Ctrl Pts',(-4.68104845693173,0.0466750239159785,
-0.0991864439809899));
#14340=CARTESIAN_POINT('Ctrl Pts',(-4.7,0.07,-0.102250208141538));
#14341=CARTESIAN_POINT('',(-4.643125,9.15359704504785E-17,0.806617578174702));
#14342=CARTESIAN_POINT('',(-4.643125,0.,1.5));
#14343=CARTESIAN_POINT('Ctrl Pts',(-4.7,0.07,0.797749791858462));
#14344=CARTESIAN_POINT('Ctrl Pts',(-4.68104845693185,0.0466750239161254,
0.800813556018989));
#14345=CARTESIAN_POINT('Ctrl Pts',(-4.66209000485925,0.0233415444421557,
0.803769188562976));
#14346=CARTESIAN_POINT('Ctrl Pts',(-4.643125,2.14053199469751E-16,0.806617578174702));
#14347=CARTESIAN_POINT('Origin',(-4.365,-0.01,3.));
#14348=CARTESIAN_POINT('',(-4.3,0.07,-0.0534076944536142));
#14349=CARTESIAN_POINT('',(-4.356875,-8.17693113320588E-17,-0.0584633454004736));
#14350=CARTESIAN_POINT('Ctrl Pts',(-4.3,0.07,-0.0534076944536142));
#14351=CARTESIAN_POINT('Ctrl Pts',(-4.31896184067339,0.046662349940442,
-0.0549913703813359));
#14352=CARTESIAN_POINT('Ctrl Pts',(-4.33792029731394,0.0233288648443822,
-0.0566762843531735));
#14353=CARTESIAN_POINT('Ctrl Pts',(-4.356875,0.,-0.0584633454004737));
#14354=CARTESIAN_POINT('',(-4.3,0.07,0.846592305546386));
#14355=CARTESIAN_POINT('',(-4.3,0.07,3.));
#14356=CARTESIAN_POINT('',(-4.356875,5.16586285118789E-16,0.841536654599526));
#14357=CARTESIAN_POINT('Ctrl Pts',(-4.356875,2.03729789587434E-16,0.841536654599527));
#14358=CARTESIAN_POINT('Ctrl Pts',(-4.33792029731394,0.0233288648443864,
0.843323715646827));
#14359=CARTESIAN_POINT('Ctrl Pts',(-4.31896184067338,0.0466623499404503,
0.845008629618665));
#14360=CARTESIAN_POINT('Ctrl Pts',(-4.3,0.07,0.846592305546386));
#14361=CARTESIAN_POINT('',(-4.356875,0.,1.5));
#14362=CARTESIAN_POINT('Origin',(-4.3,0.07,3.));
#14363=CARTESIAN_POINT('',(-4.243125,-5.25073838654019E-17,-0.0489609512621128));
#14364=CARTESIAN_POINT('Ctrl Pts',(-4.243125,0.,-0.0489609512621128));
#14365=CARTESIAN_POINT('Ctrl Pts',(-4.26208642766755,0.023337141744682,
-0.0503426355704956));
#14366=CARTESIAN_POINT('Ctrl Pts',(-4.28104488445647,0.0466706270233431,
-0.0518245802029945));
#14367=CARTESIAN_POINT('Ctrl Pts',(-4.3,0.07,-0.0534076944536142));
#14368=CARTESIAN_POINT('',(-4.243125,3.23350938624483E-16,0.851039048737887));
#14369=CARTESIAN_POINT('',(-4.243125,0.,1.5));
#14370=CARTESIAN_POINT('Ctrl Pts',(-4.3,0.07,0.846592305546386));
#14371=CARTESIAN_POINT('Ctrl Pts',(-4.28104488445647,0.0466706270233449,
0.848175419797005));
#14372=CARTESIAN_POINT('Ctrl Pts',(-4.26208642766756,0.0233371417446847,
0.849657364429504));
#14373=CARTESIAN_POINT('Ctrl Pts',(-4.243125,1.98645901944153E-16,0.851039048737887));
#14374=CARTESIAN_POINT('Origin',(-3.965,-0.01,3.));
#14375=CARTESIAN_POINT('',(-3.9,0.07,-0.0347050051502715));
#14376=CARTESIAN_POINT('',(-3.956875,4.02009657719485E-17,-0.035606825762083));
#14377=CARTESIAN_POINT('Ctrl Pts',(-3.9,0.07,-0.0347050051502715));
#14378=CARTESIAN_POINT('Ctrl Pts',(-3.91895886873206,0.04666600771439,-0.0349107717231551));
#14379=CARTESIAN_POINT('Ctrl Pts',(-3.93791732779466,0.0233325196373373,
-0.0352110736175395));
#14380=CARTESIAN_POINT('Ctrl Pts',(-3.956875,0.,-0.035606825762083));
#14381=CARTESIAN_POINT('',(-3.9,0.07,0.865294994849728));
#14382=CARTESIAN_POINT('',(-3.9,0.07,3.));
#14383=CARTESIAN_POINT('',(-3.956875,1.87037994420501E-16,0.864393174237917));
#14384=CARTESIAN_POINT('Ctrl Pts',(-3.956875,1.83482806971281E-16,0.864393174237917));
#14385=CARTESIAN_POINT('Ctrl Pts',(-3.93791732779466,0.0233325196373357,
0.86478892638246));
#14386=CARTESIAN_POINT('Ctrl Pts',(-3.91895886873206,0.0466660077143861,
0.865089228276845));
#14387=CARTESIAN_POINT('Ctrl Pts',(-3.9,0.07,0.865294994849728));
#14388=CARTESIAN_POINT('',(-3.956875,1.11022302462516E-16,1.5));
#14389=CARTESIAN_POINT('Origin',(-3.9,0.07,3.));
#14390=CARTESIAN_POINT('',(-3.843125,1.5314653627409E-16,-0.0343703987507942));
#14391=CARTESIAN_POINT('Ctrl Pts',(-3.843125,0.,-0.0343703987507941));
#14392=CARTESIAN_POINT('Ctrl Pts',(-3.86208349066526,0.0233335269726244,
-0.0343880169385557));
#14393=CARTESIAN_POINT('Ctrl Pts',(-3.88104194980522,0.046667015144881,
-0.0344992474615382));
#14394=CARTESIAN_POINT('Ctrl Pts',(-3.9,0.07,-0.0347050051502715));
#14395=CARTESIAN_POINT('',(-3.843125,2.92497646815417E-16,0.865629601249206));
#14396=CARTESIAN_POINT('',(-3.843125,0.,1.5));
#14397=CARTESIAN_POINT('Ctrl Pts',(-3.9,0.07,0.865294994849728));
#14398=CARTESIAN_POINT('Ctrl Pts',(-3.88104194980522,0.0466670151448871,
0.865500752538462));
#14399=CARTESIAN_POINT('Ctrl Pts',(-3.86208349066526,0.023333526972633,
0.865611983061444));
#14400=CARTESIAN_POINT('Ctrl Pts',(-3.843125,1.76543840779321E-16,0.865629601249206));
#14401=CARTESIAN_POINT('Origin',(-3.565,-0.01,3.));
#14402=CARTESIAN_POINT('',(-3.5,0.07,-0.044076564050104));
#14403=CARTESIAN_POINT('',(-3.556875,4.02009657719485E-17,-0.0411036357846663));
#14404=CARTESIAN_POINT('Ctrl Pts',(-3.5,0.07,-0.044076564050104));
#14405=CARTESIAN_POINT('Ctrl Pts',(-3.51895644709983,0.0466689881848213,
-0.0429970729787887));
#14406=CARTESIAN_POINT('Ctrl Pts',(-3.53791490667919,0.0233354994717666,
-0.0420057937613109));
#14407=CARTESIAN_POINT('Ctrl Pts',(-3.556875,0.,-0.0411036357846663));
#14408=CARTESIAN_POINT('',(-3.5,0.07,0.855923435949896));
#14409=CARTESIAN_POINT('',(-3.5,0.07,3.));
#14410=CARTESIAN_POINT('',(-3.556875,1.6589737310394E-16,0.858896364215334));
#14411=CARTESIAN_POINT('Ctrl Pts',(-3.556875,1.56872666502074E-16,0.858896364215334));
#14412=CARTESIAN_POINT('Ctrl Pts',(-3.53791490667898,0.0233354994720256,
0.857994206238679));
#14413=CARTESIAN_POINT('Ctrl Pts',(-3.51895644710004,0.0466689881845632,
0.857002927021225));
#14414=CARTESIAN_POINT('Ctrl Pts',(-3.5,0.07,0.855923435949896));
#14415=CARTESIAN_POINT('',(-3.556875,0.,1.5));
#14416=CARTESIAN_POINT('Origin',(-3.5,0.07,3.));
#14417=CARTESIAN_POINT('',(-3.443125,-6.56342298317527E-17,-0.0475795630490316));
#14418=CARTESIAN_POINT('Ctrl Pts',(-3.443125,0.,-0.0475795630490315));
#14419=CARTESIAN_POINT('Ctrl Pts',(-3.46208109967644,0.0233305842171503,
-0.0463242518930227));
#14420=CARTESIAN_POINT('Ctrl Pts',(-3.48103955927973,0.04666407295967,-0.0451562825418647));
#14421=CARTESIAN_POINT('Ctrl Pts',(-3.5,0.07,-0.044076564050104));
#14422=CARTESIAN_POINT('',(-3.443125,1.61329711546947E-16,0.852420436950968));
#14423=CARTESIAN_POINT('',(-3.443125,0.,1.5));
#14424=CARTESIAN_POINT('Ctrl Pts',(-3.5,0.07,0.855923435949896));
#14425=CARTESIAN_POINT('Ctrl Pts',(-3.48103955927995,0.0466640729599333,
0.854843717458145));
#14426=CARTESIAN_POINT('Ctrl Pts',(-3.46208109967623,0.023330584216898,
0.853675748106964));
#14427=CARTESIAN_POINT('Ctrl Pts',(-3.443125,1.48202865580597E-16,0.852420436950968));
#14428=CARTESIAN_POINT('Origin',(-3.165,-0.01,3.));
#14429=CARTESIAN_POINT('',(-3.1,0.07,-0.0796824742200948));
#14430=CARTESIAN_POINT('',(-3.156875,-6.83689894080757E-17,-0.0730839650446149));
#14431=CARTESIAN_POINT('Ctrl Pts',(-3.1,0.07,-0.0796824742200948));
#14432=CARTESIAN_POINT('Ctrl Pts',(-3.11895449032434,0.0466713965238894,
-0.0774003830878922));
#14433=CARTESIAN_POINT('Ctrl Pts',(-3.13791294893519,0.0233379090028467,
-0.0752005815572684));
#14434=CARTESIAN_POINT('Ctrl Pts',(-3.156875,0.,-0.0730839650446149));
#14435=CARTESIAN_POINT('',(-3.1,0.07,0.820317525779905));
#14436=CARTESIAN_POINT('',(-3.1,0.07,3.));
#14437=CARTESIAN_POINT('',(-3.156875,4.65616992992973E-16,0.826916034955385));
#14438=CARTESIAN_POINT('Ctrl Pts',(-3.156875,1.24318997867859E-16,0.826916034955385));
#14439=CARTESIAN_POINT('Ctrl Pts',(-3.13791294893498,0.0233379090031034,
0.824799418442708));
#14440=CARTESIAN_POINT('Ctrl Pts',(-3.11895449032455,0.0466713965236263,
0.822599616912135));
#14441=CARTESIAN_POINT('Ctrl Pts',(-3.1,0.07,0.820317525779905));
#14442=CARTESIAN_POINT('',(-3.156875,0.,1.5));
#14443=CARTESIAN_POINT('Origin',(-3.1,0.07,3.));
#14444=CARTESIAN_POINT('',(-3.043125,1.5314653627409E-16,-0.0867777946605038));
#14445=CARTESIAN_POINT('Ctrl Pts',(-3.043125,0.,-0.0867777946605038));
#14446=CARTESIAN_POINT('Ctrl Pts',(-3.06207917003769,0.0233282092771606,
-0.0843309193423537));
#14447=CARTESIAN_POINT('Ctrl Pts',(-3.08103762863312,0.0466616967792293,
-0.0819655142178703));
#14448=CARTESIAN_POINT('Ctrl Pts',(-3.1,0.07,-0.0796824742200948));
#14449=CARTESIAN_POINT('',(-3.043125,2.45297788588041E-16,0.813222205339496));
#14450=CARTESIAN_POINT('',(-3.043125,0.,1.5));
#14451=CARTESIAN_POINT('Ctrl Pts',(-3.1,0.07,0.820317525779905));
#14452=CARTESIAN_POINT('Ctrl Pts',(-3.08103762863333,0.0466616967794808,
0.818034485782152));
#14453=CARTESIAN_POINT('Ctrl Pts',(-3.06207917003747,0.023328209276892,
0.815669080657618));
#14454=CARTESIAN_POINT('Ctrl Pts',(-3.043125,1.14029328924536E-16,0.813222205339496));
#14455=CARTESIAN_POINT('Origin',(-2.765,-0.01,3.));
#14456=CARTESIAN_POINT('',(-2.7,0.07,-0.139875436242106));
#14457=CARTESIAN_POINT('',(-2.756875,-5.46951915264603E-17,-0.129874905216096));
#14458=CARTESIAN_POINT('Ctrl Pts',(-2.7,0.07,-0.139875436242106));
#14459=CARTESIAN_POINT('Ctrl Pts',(-2.71895292327494,0.0466733252000787,
-0.136464860017204));
#14460=CARTESIAN_POINT('Ctrl Pts',(-2.73791137978989,0.0233398402585923,
-0.133131057884513));
#14461=CARTESIAN_POINT('Ctrl Pts',(-2.756875,0.,-0.129874905216097));
#14462=CARTESIAN_POINT('',(-2.7,0.07,0.760124563757895));
#14463=CARTESIAN_POINT('',(-2.7,0.07,3.));
#14464=CARTESIAN_POINT('',(-2.756875,1.4273064411073E-17,0.770125094783904));
#14465=CARTESIAN_POINT('Ctrl Pts',(-2.756875,8.61972412683683E-17,0.770125094783903));
#14466=CARTESIAN_POINT('Ctrl Pts',(-2.73791137978969,0.0233398402588493,
0.766868942115451));
#14467=CARTESIAN_POINT('Ctrl Pts',(-2.71895292327515,0.0466733251998157,
0.763535139982836));
#14468=CARTESIAN_POINT('Ctrl Pts',(-2.7,0.07,0.760124563757895));
#14469=CARTESIAN_POINT('',(-2.756875,0.,1.5));
#14470=CARTESIAN_POINT('Origin',(-2.7,0.07,3.));
#14471=CARTESIAN_POINT('',(-2.643125,4.37561532211684E-17,-0.150342857337239));
#14472=CARTESIAN_POINT('Ctrl Pts',(-2.643125,0.,-0.150342857337239));
#14473=CARTESIAN_POINT('Ctrl Pts',(-2.6620776272105,0.0233263104129235,
-0.146777422626996));
#14474=CARTESIAN_POINT('Ctrl Pts',(-2.68103608368107,0.0466597952997781,
-0.14328799066424));
#14475=CARTESIAN_POINT('Ctrl Pts',(-2.7,0.07,-0.139875436242106));
#14476=CARTESIAN_POINT('',(-2.643125,2.12219181644668E-16,0.749657142662761));
#14477=CARTESIAN_POINT('',(-2.643125,0.,1.5));
#14478=CARTESIAN_POINT('Ctrl Pts',(-2.7,0.07,0.760124563757895));
#14479=CARTESIAN_POINT('Ctrl Pts',(-2.68103608368128,0.0466597953000397,
0.756712009335797));
#14480=CARTESIAN_POINT('Ctrl Pts',(-2.66207762721029,0.0233263104126689,
0.753222577372965));
#14481=CARTESIAN_POINT('Ctrl Pts',(-2.643125,7.43872989979874E-17,0.749657142662761));
#14482=CARTESIAN_POINT('Ctrl Pts',(-2.,0.,-0.3));
#14483=CARTESIAN_POINT('Ctrl Pts',(-4.51634900680751,0.,0.394270418819399));
#14484=CARTESIAN_POINT('Ctrl Pts',(-6.58301567347418,0.,-0.272396247847268));
#14485=CARTESIAN_POINT('Ctrl Pts',(-8.2,0.,-2.3));
#14486=CARTESIAN_POINT('Ctrl Pts',(-2.,0.333333333333333,-0.3));
#14487=CARTESIAN_POINT('Ctrl Pts',(-4.51634900680751,0.248051777551248,
0.394270418819399));
#14488=CARTESIAN_POINT('Ctrl Pts',(-6.58301567347418,0.159162888662359,
-0.272396247847267));
#14489=CARTESIAN_POINT('Ctrl Pts',(-8.2,0.0666666666666667,-2.3));
#14490=CARTESIAN_POINT('Ctrl Pts',(-2.,0.666666666666667,-0.3));
#14491=CARTESIAN_POINT('Ctrl Pts',(-4.51634900680751,0.496103555102495,
0.394270418819399));
#14492=CARTESIAN_POINT('Ctrl Pts',(-6.58301567347417,0.318325777324717,
-0.272396247847268));
#14493=CARTESIAN_POINT('Ctrl Pts',(-8.2,0.133333333333333,-2.3));
#14494=CARTESIAN_POINT('Ctrl Pts',(-2.,1.,-0.3));
#14495=CARTESIAN_POINT('Ctrl Pts',(-4.51634900680751,0.744155332653743,
0.394270418819399));
#14496=CARTESIAN_POINT('Ctrl Pts',(-6.58301567347418,0.477488665987076,
-0.272396247847268));
#14497=CARTESIAN_POINT('Ctrl Pts',(-8.2,0.2,-2.3));
#14498=CARTESIAN_POINT('Ctrl Pts',(-2.956875,0.,-0.0984757719280371));
#14499=CARTESIAN_POINT('Ctrl Pts',(-2.98568984022818,0.,-0.0943802110451274));
#14500=CARTESIAN_POINT('Ctrl Pts',(-3.01443984022818,0.,-0.090480885289283));
#14501=CARTESIAN_POINT('Ctrl Pts',(-3.043125,0.,-0.0867777946605038));
#14502=CARTESIAN_POINT('Ctrl Pts',(-3.156875,0.,-0.0730839650446149));
#14503=CARTESIAN_POINT('Ctrl Pts',(-3.18569122559797,0.,-0.0698673879599667));
#14504=CARTESIAN_POINT('Ctrl Pts',(-3.21444122559797,0.,-0.0668512387423631));
#14505=CARTESIAN_POINT('Ctrl Pts',(-3.243125,0.,-0.0640355173918041));
#14506=CARTESIAN_POINT('Ctrl Pts',(-3.356875,0.,-0.0538921790467937));
#14507=CARTESIAN_POINT('Ctrl Pts',(-3.3856926714599,0.,-0.0515831700312875));
#14508=CARTESIAN_POINT('Ctrl Pts',(-3.4144426714599,0.,-0.0494789646987002));
#14509=CARTESIAN_POINT('Ctrl Pts',(-3.443125,0.,-0.0475795630490316));
#14510=CARTESIAN_POINT('Ctrl Pts',(-3.556875,0.,-0.0411036357846664));
#14511=CARTESIAN_POINT('Ctrl Pts',(-3.58569418186451,0.,-0.0397323632724736));
#14512=CARTESIAN_POINT('Ctrl Pts',(-3.61444418186451,0.,-0.0385704655936833));
#14513=CARTESIAN_POINT('Ctrl Pts',(-3.643125,0.,-0.0376179427482956));
#14514=CARTESIAN_POINT('Ctrl Pts',(-3.756875,0.,-0.0349329077078822));
#14515=CARTESIAN_POINT('Ctrl Pts',(-3.78569576123222,0.,-0.034531250025529));
#14516=CARTESIAN_POINT('Ctrl Pts',(-3.81444576123222,0.,-0.034343747039833));
#14517=CARTESIAN_POINT('Ctrl Pts',(-3.843125,0.,-0.0343703987507942));
#14518=CARTESIAN_POINT('Ctrl Pts',(-3.956875,0.,-0.035606825762083));
#14519=CARTESIAN_POINT('Ctrl Pts',(-3.98569741439656,0.,-0.0362085099870666));
#14520=CARTESIAN_POINT('Ctrl Pts',(-4.01444741439656,0.,-0.0370293521131091));
#14521=CARTESIAN_POINT('Ctrl Pts',(-4.043125,0.,-0.0380693521402107));
#14522=CARTESIAN_POINT('Ctrl Pts',(-4.156875,0.,-0.0433654828435956));
#14523=CARTESIAN_POINT('Ctrl Pts',(-4.18569914665357,0.,-0.0450062385083631));
#14524=CARTESIAN_POINT('Ctrl Pts',(-4.21444914665357,0.,-0.0468713946478688));
#14525=CARTESIAN_POINT('Ctrl Pts',(-4.243125,0.,-0.0489609512621128));
#14526=CARTESIAN_POINT('Ctrl Pts',(-4.356875,0.,-0.0584633454004736));
#14527=CARTESIAN_POINT('Ctrl Pts',(-4.38570096381845,0.,-0.0611810750290543));
#14528=CARTESIAN_POINT('Ctrl Pts',(-4.41445096381845,0.,-0.064128704674742));
#14529=CARTESIAN_POINT('Ctrl Pts',(-4.443125,0.,-0.0673062343375367));
#14530=CARTESIAN_POINT('Ctrl Pts',(-4.556875,0.,-0.0811704877759833));
#14531=CARTESIAN_POINT('Ctrl Pts',(-4.58570287229084,0.,-0.0850054565628438));
#14532=CARTESIAN_POINT('Ctrl Pts',(-4.61445287229084,0.,-0.0890761012459485));
#14533=CARTESIAN_POINT('Ctrl Pts',(-4.643125,0.,-0.0933824218252977));
#14534=CARTESIAN_POINT('Ctrl Pts',(-4.756875,0.,-0.11177396627754));
#14535=CARTESIAN_POINT('Ctrl Pts',(-4.78570487913006,0.,-0.116769013602367));
#14536=CARTESIAN_POINT('Ctrl Pts',(-4.81445487913006,0.,-0.122005810403998));
#14537=CARTESIAN_POINT('Ctrl Pts',(-4.843125,0.,-0.127484356682433));
#14538=CARTESIAN_POINT('Ctrl Pts',(-4.956875,0.,-0.150579352803062));
#14539=CARTESIAN_POINT('Ctrl Pts',(-4.98570699214241,0.,-0.156780128734979));
#14540=CARTESIAN_POINT('Ctrl Pts',(-5.01445699214242,0.,-0.163229049050992));
#14541=CARTESIAN_POINT('Ctrl Pts',(-5.043125,0.,-0.169926113751101));
#14542=CARTESIAN_POINT('Ctrl Pts',(-5.156875,0.,-0.197912451271776));
#14543=CARTESIAN_POINT('Ctrl Pts',(-5.18570921998266,0.,-0.205367681769314));
#14544=CARTESIAN_POINT('Ctrl Pts',(-5.21445921998266,0.,-0.213077799078072));
#14545=CARTESIAN_POINT('Ctrl Pts',(-5.243125,0.,-0.221042803198049));
#14546=CARTESIAN_POINT('Ctrl Pts',(-5.356875,0.,-0.25412122421867));
#14547=CARTESIAN_POINT('Ctrl Pts',(-5.38571157227249,0.,-0.262883009399545));
#14548=CARTESIAN_POINT('Ctrl Pts',(-5.41446157227249,0.,-0.271906800458094));
#14549=CARTESIAN_POINT('Ctrl Pts',(-5.443125,0.,-0.281192597394316));
#14550=CARTESIAN_POINT('Ctrl Pts',(-5.556875,0.,-0.319577961886773));
#14551=CARTESIAN_POINT('Ctrl Pts',(-5.58571405973946,0.,-0.329702112552068));
#14552=CARTESIAN_POINT('Ctrl Pts',(-5.61446405973946,0.,-0.340095797267151));
#14553=CARTESIAN_POINT('Ctrl Pts',(-5.643125,0.,-0.350759016032021));
#14554=CARTESIAN_POINT('Ctrl Pts',(-5.756875,0.,-0.394681732200484));
#14555=CARTESIAN_POINT('Ctrl Pts',(-5.78571669438059,0.,-0.406228150786744));
#14556=CARTESIAN_POINT('Ctrl Pts',(-5.81446669438059,0.,-0.418052077008794));
#14557=CARTESIAN_POINT('Ctrl Pts',(-5.843125,0.,-0.430153510866633));
#14558=CARTESIAN_POINT('Ctrl Pts',(-5.956875,0.,-0.479861157396718));
#14559=CARTESIAN_POINT('Ctrl Pts',(-5.98571948965581,0.,-0.492894270742694));
#14560=CARTESIAN_POINT('Ctrl Pts',(-6.01446948965581,0.,-0.506213351460083));
#14561=CARTESIAN_POINT('Ctrl Pts',(-6.043125,0.,-0.519818399548886));
#14562=CARTESIAN_POINT('Ctrl Pts',(-6.156875,0.,-0.575577572177906));
#14563=CARTESIAN_POINT('Ctrl Pts',(-6.18572246071802,0.,-0.590166824989555));
#14564=CARTESIAN_POINT('Ctrl Pts',(-6.21447246071802,0.,-0.60505103691722));
#14565=CARTESIAN_POINT('Ctrl Pts',(-6.243125,0.,-0.620230207960902));
#14566=CARTESIAN_POINT('Ctrl Pts',(-6.356875,0.,-0.682328629485448));
#14567=CARTESIAN_POINT('Ctrl Pts',(-6.3857256246879,0.,-0.698549049241059));
#14568=CARTESIAN_POINT('Ctrl Pts',(-6.4144756246879,0.,-0.715074003680945));
#14569=CARTESIAN_POINT('Ctrl Pts',(-6.443125,0.,-0.731903492805105));
#14570=CARTESIAN_POINT('Ctrl Pts',(-6.556875,0.,-0.800652433967885));
#14571=CARTESIAN_POINT('Ctrl Pts',(-6.585729000984,0.,-0.818585280326885));
#14572=CARTESIAN_POINT('Ctrl Pts',(-6.614479000984,0.,-0.836832879531224));
#14573=CARTESIAN_POINT('Ctrl Pts',(-6.643125,0.,-0.8553952315809));
#14574=CARTESIAN_POINT('Ctrl Pts',(-6.756875,0.,-0.93113230071851));
#14575=CARTESIAN_POINT('Ctrl Pts',(-6.78573261172172,0.,-0.950865815418223));
#14576=CARTESIAN_POINT('Ctrl Pts',(-6.81448261172172,0.,-0.970925010648066));
#14577=CARTESIAN_POINT('Ctrl Pts',(-6.843125,0.,-0.991309886408041));
#14578=CARTESIAN_POINT('Ctrl Pts',(-6.956875,0.,-1.07440225892494));
#14579=CARTESIAN_POINT('Ctrl Pts',(-6.98573648219828,0.,-1.09603253585073));
#14580=CARTESIAN_POINT('Ctrl Pts',(-7.01448648219828,0.,-1.11800020707571));
#14581=CARTESIAN_POINT('Ctrl Pts',(-7.043125,0.,-1.14030527259989));
#14582=CARTESIAN_POINT('Ctrl Pts',(-7.156875,0.,-1.23115344810839));
#14583=CARTESIAN_POINT('Ctrl Pts',(-7.18574064148632,0.,-1.25478544794926));
#14584=CARTESIAN_POINT('Ctrl Pts',(-7.21449064148632,0.,-1.27876742992929));
#14585=CARTESIAN_POINT('Ctrl Pts',(-7.243125,0.,-1.3030993940485));
#14586=CARTESIAN_POINT('Ctrl Pts',(-7.356875,0.,-1.40214159053033));
#14587=CARTESIAN_POINT('Ctrl Pts',(-7.38574512316552,0.,-1.42789033051882));
#14588=CARTESIAN_POINT('Ctrl Pts',(-7.41449512316552,0.,-1.45400261618429));
#14589=CARTESIAN_POINT('Ctrl Pts',(-7.443125,0.,-1.48047844752676));
#14590=CARTESIAN_POINT('Ctrl Pts',(-7.556875,0.,-1.58819576970747));
#14591=CARTESIAN_POINT('Ctrl Pts',(-7.58574996623124,0.,-1.61618772685047));
#14592=CARTESIAN_POINT('Ctrl Pts',(-7.61449996623124,0.,-1.64455788692328));
#14593=CARTESIAN_POINT('Ctrl Pts',(-7.643125,0.,-1.67330624992589));
#14594=CARTESIAN_POINT('Ctrl Pts',(-7.756875,0.,-1.79022880539828));
#14595=CARTESIAN_POINT('Ctrl Pts',(-7.78575521623218,0.,-1.82060358197814));
#14596=CARTESIAN_POINT('Ctrl Pts',(-7.81450521623218,0.,-1.85137245030608));
#14597=CARTESIAN_POINT('Ctrl Pts',(-7.843125,0.,-1.8825354103821));
#14598=CARTESIAN_POINT('',(-8.2,0.,-2.3));
#14599=CARTESIAN_POINT('Ctrl Pts',(-7.956875,0.,-2.0092495949436));
#14600=CARTESIAN_POINT('Ctrl Pts',(-8.03901579912867,0.,-2.10283993704666));
#14601=CARTESIAN_POINT('Ctrl Pts',(-8.12005746579533,0.,-2.19975673873213));
#14602=CARTESIAN_POINT('Ctrl Pts',(-8.2,0.,-2.3));
#14603=CARTESIAN_POINT('',(-8.2,0.2,-2.3));
#14604=CARTESIAN_POINT('',(-8.2,0.,-2.3));
#14605=CARTESIAN_POINT('',(-2.,1.,-0.3));
#14606=CARTESIAN_POINT('Ctrl Pts',(-2.,1.,-0.3));
#14607=CARTESIAN_POINT('Ctrl Pts',(-3.28369393227907,0.869483030299115,
0.0541761184908199));
#14608=CARTESIAN_POINT('Ctrl Pts',(-4.45036059894574,0.736149696965781,
0.0541761184908199));
#14609=CARTESIAN_POINT('Ctrl Pts',(-6.50790640323229,0.469263528758431,
-0.640094300328579));
#14610=CARTESIAN_POINT('Ctrl Pts',(-7.40790640323229,0.335930195425098,
-1.30676096699525));
#14611=CARTESIAN_POINT('Ctrl Pts',(-8.2,0.2,-2.3));
#14612=CARTESIAN_POINT('',(-2.,0.,-0.3));
#14613=CARTESIAN_POINT('',(-2.,0.,-0.3));
#14614=CARTESIAN_POINT('Ctrl Pts',(-2.,0.,-0.3));
#14615=CARTESIAN_POINT('Ctrl Pts',(-2.21774204304033,0.,-0.239924128565937));
#14616=CARTESIAN_POINT('Ctrl Pts',(-2.43211704304033,0.,-0.190038414345017));
#14617=CARTESIAN_POINT('Ctrl Pts',(-2.643125,0.,-0.150342857337239));
#14618=CARTESIAN_POINT('Ctrl Pts',(-2.756875,0.,-0.129874905216096));
#14619=CARTESIAN_POINT('Ctrl Pts',(-2.78568851163198,0.,-0.124927474728276));
#14620=CARTESIAN_POINT('Ctrl Pts',(-2.81443851163198,0.,-0.120172258449476));
#14621=CARTESIAN_POINT('Ctrl Pts',(-2.843125,0.,-0.115609256379697));
#14622=CARTESIAN_POINT('Origin',(-2.,0.,0.));
#14623=CARTESIAN_POINT('',(-8.2,-5.55111512312578E-17,-1.4));
#14624=CARTESIAN_POINT('Ctrl Pts',(-7.956875,-5.68405272773173E-18,-1.1092495949436));
#14625=CARTESIAN_POINT('Ctrl Pts',(-8.03901579912867,-2.14768189374877E-17,
-1.20283993704666));
#14626=CARTESIAN_POINT('Ctrl Pts',(-8.12005746579533,-3.80858517719964E-17,
-1.29975673873213));
#14627=CARTESIAN_POINT('Ctrl Pts',(-8.2,-5.55111512312578E-17,-1.4));
#14628=CARTESIAN_POINT('',(-8.2,0.,-1.4));
#14629=CARTESIAN_POINT('Origin',(-2.,0.,0.));
#14630=CARTESIAN_POINT('',(-2.,0.,0.));
#14631=CARTESIAN_POINT('',(-2.,0.,0.6));
#14632=CARTESIAN_POINT('',(-1.4,0.,0.));
#14633=CARTESIAN_POINT('',(-1.2,0.,0.));
#14634=CARTESIAN_POINT('',(-1.4,0.,0.6));
#14635=CARTESIAN_POINT('',(-1.4,0.,0.));
#14636=CARTESIAN_POINT('',(-2.,0.,0.6));
#14637=CARTESIAN_POINT('',(-1.2,0.,0.6));
#14638=CARTESIAN_POINT('Ctrl Pts',(-2.,0.,0.6));
#14639=CARTESIAN_POINT('Ctrl Pts',(-2.21774204304033,2.72962882924285E-17,
0.660075871434063));
#14640=CARTESIAN_POINT('Ctrl Pts',(-2.43211704304033,5.2092054625091E-17,
0.709961585654983));
#14641=CARTESIAN_POINT('Ctrl Pts',(-2.643125,7.43872989979873E-17,0.749657142662761));
#14642=CARTESIAN_POINT('Origin',(-2.,0.,0.));
#14643=CARTESIAN_POINT('Ctrl Pts',(-2.956875,1.05932212640155E-16,0.801524228071963));
#14644=CARTESIAN_POINT('Ctrl Pts',(-2.98568984022818,1.08679404755311E-16,
0.805619788954873));
#14645=CARTESIAN_POINT('Ctrl Pts',(-3.01443984022818,1.11378443516772E-16,
0.809519114710717));
#14646=CARTESIAN_POINT('Ctrl Pts',(-3.043125,1.14029328924536E-16,0.813222205339496));
#14647=CARTESIAN_POINT('Origin',(-2.,0.,0.));
#14648=CARTESIAN_POINT('Ctrl Pts',(-3.356875,1.41314351751907E-16,0.846107820953206));
#14649=CARTESIAN_POINT('Ctrl Pts',(-3.3856926714599,1.43660778985515E-16,
0.848416829968713));
#14650=CARTESIAN_POINT('Ctrl Pts',(-3.4144426714599,1.45956950261745E-16,
0.8505210353013));
#14651=CARTESIAN_POINT('Ctrl Pts',(-3.443125,1.48202865580597E-16,0.852420436950969));
#14652=CARTESIAN_POINT('Origin',(-2.,0.,0.));
#14653=CARTESIAN_POINT('Ctrl Pts',(-3.756875,1.70945786985105E-16,0.865067092292118));
#14654=CARTESIAN_POINT('Ctrl Pts',(-3.78569576123222,1.72864355481784E-16,
0.865468749974471));
#14655=CARTESIAN_POINT('Ctrl Pts',(-3.81444576123222,1.74730373413189E-16,
0.865656252960167));
#14656=CARTESIAN_POINT('Ctrl Pts',(-3.843125,1.76543840779321E-16,0.865629601249206));
#14657=CARTESIAN_POINT('Origin',(-2.,0.,0.));
#14658=CARTESIAN_POINT('Ctrl Pts',(-4.156875,1.94429843935443E-16,0.856634517156404));
#14659=CARTESIAN_POINT('Ctrl Pts',(-4.18569914665357,1.95890261340829E-16,
0.854993761491637));
#14660=CARTESIAN_POINT('Ctrl Pts',(-4.21444914665357,1.97295614010399E-16,
0.853128605352131));
#14661=CARTESIAN_POINT('Ctrl Pts',(-4.243125,1.98645901944153E-16,0.851039048737887));
#14662=CARTESIAN_POINT('Origin',(-2.,0.,0.));
#14663=CARTESIAN_POINT('Ctrl Pts',(-4.556875,2.11322032856213E-16,0.818829512224017));
#14664=CARTESIAN_POINT('Ctrl Pts',(-4.58570287229084,2.12290253293836E-16,
0.814994543437156));
#14665=CARTESIAN_POINT('Ctrl Pts',(-4.61445287229084,2.13200642165015E-16,
0.810923898754051));
#14666=CARTESIAN_POINT('Ctrl Pts',(-4.643125,2.14053199469751E-16,0.806617578174702));
#14667=CARTESIAN_POINT('Origin',(-2.,0.,0.));
#14668=CARTESIAN_POINT('Ctrl Pts',(-4.956875,2.211215680057E-16,0.749420647196938));
#14669=CARTESIAN_POINT('Ctrl Pts',(-4.98570699214242,2.21559106727351E-16,
0.743219871265021));
#14670=CARTESIAN_POINT('Ctrl Pts',(-5.01445699214242,2.21935754290147E-16,
0.736770950949008));
#14671=CARTESIAN_POINT('Ctrl Pts',(-5.043125,2.22251510694088E-16,0.730073886248898));
#14672=CARTESIAN_POINT('Origin',(-2.,0.,0.));
#14673=CARTESIAN_POINT('Ctrl Pts',(-5.156875,2.23187164218309E-16,0.702087548728224));
#14674=CARTESIAN_POINT('Ctrl Pts',(-5.18570921998266,2.23343314999352E-16,
0.694632318230686));
#14675=CARTESIAN_POINT('Ctrl Pts',(-5.21445921998266,2.2343692012429E-16,
0.686922200921928));
#14676=CARTESIAN_POINT('Ctrl Pts',(-5.243125,2.23467979593124E-16,0.678957196801952));
#14677=CARTESIAN_POINT('Origin',(-2.,0.,0.));
#14678=CARTESIAN_POINT('Ctrl Pts',(-5.556875,2.21259072005402E-16,0.580422038113227));
#14679=CARTESIAN_POINT('Ctrl Pts',(-5.58571405973946,2.20816561009998E-16,
0.570297887447932));
#14680=CARTESIAN_POINT('Ctrl Pts',(-5.61446405973946,2.20307910131147E-16,
0.559904202732849));
#14681=CARTESIAN_POINT('Ctrl Pts',(-5.643125,2.19733119368846E-16,0.549240983967979));
#14682=CARTESIAN_POINT('Origin',(-2.,0.,0.));
#14683=CARTESIAN_POINT('Ctrl Pts',(-5.956875,2.10664257829173E-16,0.420138842603282));
#14684=CARTESIAN_POINT('Ctrl Pts',(-5.98571948965581,2.09569251279892E-16,
0.407105729257306));
#14685=CARTESIAN_POINT('Ctrl Pts',(-6.01446948965581,2.08404072340035E-16,
0.393786648539917));
#14686=CARTESIAN_POINT('Ctrl Pts',(-6.043125,2.07168721009601E-16,0.380181600451114));
#14687=CARTESIAN_POINT('Origin',(-2.,0.,0.));
#14688=CARTESIAN_POINT('Ctrl Pts',(-6.356875,1.90602294150671E-16,0.217671370514552));
#14689=CARTESIAN_POINT('Ctrl Pts',(-6.3857256246879,1.8879236986419E-16,
0.201450950758941));
#14690=CARTESIAN_POINT('Ctrl Pts',(-6.4144756246879,1.86907717028423E-16,
0.184925996319055));
#14691=CARTESIAN_POINT('Ctrl Pts',(-6.443125,1.84948335643369E-16,0.168096507194894));
#14692=CARTESIAN_POINT('Origin',(-2.,0.,0.));
#14693=CARTESIAN_POINT('Ctrl Pts',(-6.756875,1.60141391335515E-16,-0.0311323007185111));
#14694=CARTESIAN_POINT('Ctrl Pts',(-6.78573261172172,1.57543488710523E-16,
-0.0508658154182241));
#14695=CARTESIAN_POINT('Ctrl Pts',(-6.81448261172172,1.54865668641626E-16,
-0.070925010648067));
#14696=CARTESIAN_POINT('Ctrl Pts',(-6.843125,1.52107931128825E-16,-0.0913098864080408));
#14697=CARTESIAN_POINT('Origin',(-2.,0.,0.));
#14698=CARTESIAN_POINT('Ctrl Pts',(-7.156875,1.18186075359093E-16,-0.331153448108389));
#14699=CARTESIAN_POINT('Ctrl Pts',(-7.18574064148632,1.14713769871462E-16,
-0.354785447949256));
#14700=CARTESIAN_POINT('Ctrl Pts',(-7.21449064148632,1.1115558366519E-16,
-0.378767429929292));
#14701=CARTESIAN_POINT('Ctrl Pts',(-7.243125,1.07511516740278E-16,-0.403099394048499));
#14702=CARTESIAN_POINT('Origin',(-2.,0.,0.));
#14703=CARTESIAN_POINT('Ctrl Pts',(-7.556875,6.34338590962456E-17,-0.688195769707468));
#14704=CARTESIAN_POINT('Ctrl Pts',(-7.58574996623124,5.89836676325215E-17,
-0.716187726850472));
#14705=CARTESIAN_POINT('Ctrl Pts',(-7.61449996623124,5.44406704631115E-17,
-0.744557886923278));
#14706=CARTESIAN_POINT('Ctrl Pts',(-7.643125,4.98048675880153E-17,-0.773306249925886));
#14707=CARTESIAN_POINT('Origin',(-2.,0.,0.));
#14708=CARTESIAN_POINT('Ctrl Pts',(-7.356875,9.25005547396036E-17,-0.502141590530332));
#14709=CARTESIAN_POINT('Ctrl Pts',(-7.38574512316552,8.85534870165421E-17,
-0.527890330518817));
#14710=CARTESIAN_POINT('Ctrl Pts',(-7.41449512316552,8.45172102724934E-17,
-0.554002616184292));
#14711=CARTESIAN_POINT('Ctrl Pts',(-7.443125,8.03917245074572E-17,-0.580478447526758));
#14712=CARTESIAN_POINT('Origin',(-2.,0.,0.));
#14713=CARTESIAN_POINT('Ctrl Pts',(-6.956875,1.4067648690722E-16,-0.174402258924943));
#14714=CARTESIAN_POINT('Ctrl Pts',(-6.98573648219828,1.37653151520309E-16,
-0.196032535850728));
#14715=CARTESIAN_POINT('Ctrl Pts',(-7.01448648219828,1.34547024294509E-16,
-0.21800020707571));
#14716=CARTESIAN_POINT('Ctrl Pts',(-7.043125,1.3135810522982E-16,-0.240305272599889));
#14717=CARTESIAN_POINT('Origin',(-2.,0.,0.));
#14718=CARTESIAN_POINT('Ctrl Pts',(-6.556875,1.76735896700934E-16,0.0993475660321151));
#14719=CARTESIAN_POINT('Ctrl Pts',(-6.585729000984,1.74541877575129E-16,
0.0814147196731151));
#14720=CARTESIAN_POINT('Ctrl Pts',(-6.614479000984,1.72270622506326E-16,
0.0631671204687766));
#14721=CARTESIAN_POINT('Ctrl Pts',(-6.643125,1.69922131494523E-16,0.0446047684190991));
#14722=CARTESIAN_POINT('Origin',(-2.,0.,0.));
#14723=CARTESIAN_POINT('Ctrl Pts',(-6.156875,2.0187149338955E-16,0.324422427822094));
#14724=CARTESIAN_POINT('Ctrl Pts',(-6.18572246071802,2.00427440822935E-16,
0.309833175010445));
#14725=CARTESIAN_POINT('Ctrl Pts',(-6.21447246071802,1.98911009417466E-16,
0.294948963082779));
#14726=CARTESIAN_POINT('Ctrl Pts',(-6.243125,1.97322199173142E-16,0.279769792039098));
#14727=CARTESIAN_POINT('Origin',(-2.,0.,0.));
#14728=CARTESIAN_POINT('Ctrl Pts',(-5.756875,2.17092272561204E-16,0.505318267799516));
#14729=CARTESIAN_POINT('Ctrl Pts',(-5.78571669438058,2.16330738146735E-16,
0.493771849213256));
#14730=CARTESIAN_POINT('Ctrl Pts',(-5.81446669438058,2.15501107242411E-16,
0.481947922991206));
#14731=CARTESIAN_POINT('Ctrl Pts',(-5.843125,2.1460337984823E-16,0.469846489133367));
#14732=CARTESIAN_POINT('Origin',(-2.,0.,0.));
#14733=CARTESIAN_POINT('Ctrl Pts',(-5.356875,2.23260849130472E-16,0.64587877578133));
#14734=CARTESIAN_POINT('Ctrl Pts',(-5.38571157227249,2.23123927367347E-16,
0.637116990600455));
#14735=CARTESIAN_POINT('Ctrl Pts',(-5.41446157227249,2.22922713028847E-16,
0.628093199541906));
#14736=CARTESIAN_POINT('Ctrl Pts',(-5.443125,2.22657206114972E-16,0.618807402605684));
#14737=CARTESIAN_POINT('Origin',(-2.,0.,0.));
#14738=CARTESIAN_POINT('Ctrl Pts',(-7.756875,3.0781130083136E-17,-0.890228805398279));
#14739=CARTESIAN_POINT('Ctrl Pts',(-7.78575521623218,2.57965106409104E-17,
-0.920603581978137));
#14740=CARTESIAN_POINT('Ctrl Pts',(-7.81450521623218,2.07151865993711E-17,
-0.951372450306077));
#14741=CARTESIAN_POINT('Ctrl Pts',(-7.843125,1.55371579585189E-17,-0.982535410382095));
#14742=CARTESIAN_POINT('Origin',(-2.,0.,0.));
#14743=CARTESIAN_POINT('Ctrl Pts',(-4.756875,2.17142151516292E-16,0.78822603372246));
#14744=CARTESIAN_POINT('Ctrl Pts',(-4.78570487913006,2.17850150205713E-16,
0.783230986397633));
#14745=CARTESIAN_POINT('Ctrl Pts',(-4.81445487913006,2.18498826957025E-16,
0.777994189596002));
#14746=CARTESIAN_POINT('Ctrl Pts',(-4.843125,2.19088181770229E-16,0.772515643317567));
#14747=CARTESIAN_POINT('Origin',(-2.,0.,0.));
#14748=CARTESIAN_POINT('Ctrl Pts',(-4.356875,2.03729789587434E-16,0.841536654599527));
#14749=CARTESIAN_POINT('Ctrl Pts',(-4.38570096381846,2.04948623843645E-16,
0.838818924970946));
#14750=CARTESIAN_POINT('Ctrl Pts',(-4.41445096381846,2.06111043853314E-16,
0.835871295325259));
#14751=CARTESIAN_POINT('Ctrl Pts',(-4.443125,2.07217049616441E-16,0.832693765662464));
#14752=CARTESIAN_POINT('Origin',(-2.,0.,0.));
#14753=CARTESIAN_POINT('Ctrl Pts',(-3.956875,1.83482806971281E-16,0.864393174237917));
#14754=CARTESIAN_POINT('Ctrl Pts',(-3.98569741439656,1.8517630668956E-16,
0.863791490012933));
#14755=CARTESIAN_POINT('Ctrl Pts',(-4.01444741439656,1.8681602812623E-16,
0.862970647886891));
#14756=CARTESIAN_POINT('Ctrl Pts',(-4.043125,1.88401971281291E-16,0.861930647859789));
#14757=CARTESIAN_POINT('Origin',(-2.,0.,0.));
#14758=CARTESIAN_POINT('Ctrl Pts',(-3.556875,1.56872666502074E-16,0.858896364215334));
#14759=CARTESIAN_POINT('Ctrl Pts',(-3.58569418186451,1.59008739304927E-16,
0.860267636727527));
#14760=CARTESIAN_POINT('Ctrl Pts',(-3.61444418186451,1.61093434454052E-16,
0.861429534406317));
#14761=CARTESIAN_POINT('Ctrl Pts',(-3.643125,1.63126751949447E-16,0.862382057251704));
#14762=CARTESIAN_POINT('Origin',(-2.,0.,0.));
#14763=CARTESIAN_POINT('Ctrl Pts',(-3.156875,1.24318997867859E-16,0.826916034955385));
#14764=CARTESIAN_POINT('Ctrl Pts',(-3.18569122559797,1.26869013116654E-16,
0.830132612040033));
#14765=CARTESIAN_POINT('Ctrl Pts',(-3.21444122559797,1.29369846172042E-16,
0.833148761257637));
#14766=CARTESIAN_POINT('Ctrl Pts',(-3.243125,1.31821497034025E-16,0.835964482608196));
#14767=CARTESIAN_POINT('Origin',(-8.2,0.1,-1.85));
#14768=CARTESIAN_POINT('',(-8.2,0.2,-1.4));
#14769=CARTESIAN_POINT('',(-8.2,0.2,-1.4));
#14770=CARTESIAN_POINT('',(-8.2,0.2,-2.3));
#14771=CARTESIAN_POINT('Origin',(-2.,0.5,0.15));
#14772=CARTESIAN_POINT('',(-2.,1.,0.));
#14773=CARTESIAN_POINT('',(-2.,0.,0.));
#14774=CARTESIAN_POINT('',(-2.,1.,-0.3));
#14775=CARTESIAN_POINT('Ctrl Pts',(-2.,1.,-0.3));
#14776=CARTESIAN_POINT('Ctrl Pts',(-4.51634900680751,0.744155332653743,
0.394270418819399));
#14777=CARTESIAN_POINT('Ctrl Pts',(-6.58301567347418,0.477488665987076,
-0.272396247847268));
#14778=CARTESIAN_POINT('Ctrl Pts',(-8.2,0.2,-2.3));
#14779=CARTESIAN_POINT('Ctrl Pts',(-2.,1.,-5.55111512312578E-17));
#14780=CARTESIAN_POINT('Ctrl Pts',(-4.51634900680751,0.744155332653743,
0.694270418819399));
#14781=CARTESIAN_POINT('Ctrl Pts',(-6.58301567347418,0.477488665987076,
0.027603752152733));
#14782=CARTESIAN_POINT('Ctrl Pts',(-8.2,0.2,-2.));
#14783=CARTESIAN_POINT('Ctrl Pts',(-2.,1.,0.3));
#14784=CARTESIAN_POINT('Ctrl Pts',(-4.51634900680751,0.744155332653743,
0.994270418819399));
#14785=CARTESIAN_POINT('Ctrl Pts',(-6.58301567347417,0.477488665987077,
0.327603752152732));
#14786=CARTESIAN_POINT('Ctrl Pts',(-8.2,0.2,-1.7));
#14787=CARTESIAN_POINT('Ctrl Pts',(-2.,1.,0.6));
#14788=CARTESIAN_POINT('Ctrl Pts',(-4.51634900680751,0.744155332653743,
1.2942704188194));
#14789=CARTESIAN_POINT('Ctrl Pts',(-6.58301567347418,0.477488665987076,
0.627603752152732));
#14790=CARTESIAN_POINT('Ctrl Pts',(-8.2,0.2,-1.4));
#14791=CARTESIAN_POINT('',(-2.,1.,0.6));
#14792=CARTESIAN_POINT('Ctrl Pts',(-2.,1.,0.6));
#14793=CARTESIAN_POINT('Ctrl Pts',(-3.28369393227907,0.869483030299115,
0.95417611849082));
#14794=CARTESIAN_POINT('Ctrl Pts',(-4.45036059894574,0.736149696965781,
0.95417611849082));
#14795=CARTESIAN_POINT('Ctrl Pts',(-6.50790640323229,0.469263528758431,
0.259905699671421));
#14796=CARTESIAN_POINT('Ctrl Pts',(-7.40790640323229,0.335930195425098,
-0.406760966995246));
#14797=CARTESIAN_POINT('Ctrl Pts',(-8.2,0.2,-1.4));
#14798=CARTESIAN_POINT('',(-2.,1.,0.));
#14799=CARTESIAN_POINT('Ctrl Pts',(-2.,1.,0.6));
#14800=CARTESIAN_POINT('Ctrl Pts',(-4.51634900680751,0.744155332653743,
1.2942704188194));
#14801=CARTESIAN_POINT('Ctrl Pts',(-6.58301567347418,0.477488665987076,
0.627603752152733));
#14802=CARTESIAN_POINT('Ctrl Pts',(-8.2,0.2,-1.4));
#14803=CARTESIAN_POINT('Ctrl Pts',(-2.,0.666666666666667,0.6));
#14804=CARTESIAN_POINT('Ctrl Pts',(-4.51634900680751,0.496103555102495,
1.2942704188194));
#14805=CARTESIAN_POINT('Ctrl Pts',(-6.58301567347418,0.318325777324718,
0.627603752152732));
#14806=CARTESIAN_POINT('Ctrl Pts',(-8.2,0.133333333333333,-1.4));
#14807=CARTESIAN_POINT('Ctrl Pts',(-2.,0.333333333333333,0.6));
#14808=CARTESIAN_POINT('Ctrl Pts',(-4.51634900680751,0.248051777551248,
1.2942704188194));
#14809=CARTESIAN_POINT('Ctrl Pts',(-6.58301567347417,0.159162888662359,
0.627603752152733));
#14810=CARTESIAN_POINT('Ctrl Pts',(-8.2,0.0666666666666667,-1.4));
#14811=CARTESIAN_POINT('Ctrl Pts',(-2.,0.,0.6));
#14812=CARTESIAN_POINT('Ctrl Pts',(-4.51634900680751,3.15451196172815E-16,
1.2942704188194));
#14813=CARTESIAN_POINT('Ctrl Pts',(-6.58301567347418,2.96947479095729E-16,
0.627603752152733));
#14814=CARTESIAN_POINT('Ctrl Pts',(-8.2,-5.55111512312578E-17,-1.4));
#14815=CARTESIAN_POINT('Ctrl Pts',(-2.756875,8.61972412683683E-17,0.770125094783904));
#14816=CARTESIAN_POINT('Ctrl Pts',(-2.78568851163198,8.91355287853243E-17,
0.775072525271724));
#14817=CARTESIAN_POINT('Ctrl Pts',(-2.81443851163198,9.20266496255957E-17,
0.779827741550524));
#14818=CARTESIAN_POINT('Ctrl Pts',(-2.843125,9.48706037891828E-17,0.784390743620303));
#14819=CARTESIAN_POINT('',(-2.,0.,0.6));
#14820=CARTESIAN_POINT('Origin',(-2.,0.,0.));
#14821=CARTESIAN_POINT('Origin',(-1.2,1.,0.));
#14822=CARTESIAN_POINT('',(-1.2,1.,0.));
#14823=CARTESIAN_POINT('',(-2.,1.,0.));
#14824=CARTESIAN_POINT('',(-1.2,1.,0.6));
#14825=CARTESIAN_POINT('',(-2.,1.,0.6));
#14826=CARTESIAN_POINT('',(-1.2,1.,0.));
#14827=CARTESIAN_POINT('Origin',(-1.2,0.,0.));
#14828=CARTESIAN_POINT('',(-1.2,0.721110255092798,0.));
#14829=CARTESIAN_POINT('',(-1.2,0.721110255092798,0.6));
#14830=CARTESIAN_POINT('',(-1.2,0.721110255092798,0.));
#14831=CARTESIAN_POINT('',(-1.2,1.,0.));
#14832=CARTESIAN_POINT('',(-1.2,1.,0.6));
#14833=CARTESIAN_POINT('Origin',(0.,0.,0.));
#14834=CARTESIAN_POINT('',(0.533017816115691,-1.29456247732709,0.));
#14835=CARTESIAN_POINT('Origin',(0.,0.,0.));
#14836=CARTESIAN_POINT('',(0.533017816115691,-1.29456247732709,0.6));
#14837=CARTESIAN_POINT('',(0.533017816115691,-1.29456247732709,0.));
#14838=CARTESIAN_POINT('Origin',(0.,0.,0.6));
#14839=CARTESIAN_POINT('Origin',(0.,0.,0.));
#14840=CARTESIAN_POINT('',(0.993295878967653,0.986591757935306,0.6));
#14841=CARTESIAN_POINT('Origin',(0.,0.,0.6));
#14842=CARTESIAN_POINT('',(0.993295878967653,0.986591757935306,0.));
#14843=CARTESIAN_POINT('',(0.993295878967653,0.986591757935306,0.));
#14844=CARTESIAN_POINT('Origin',(0.,0.,0.));
#14845=CARTESIAN_POINT('Origin',(0.,0.,0.6));
#14846=CARTESIAN_POINT('',(3.8,-3.1,0.6));
#14847=CARTESIAN_POINT('',(0.,-1.,0.6));
#14848=CARTESIAN_POINT('',(14.,-3.1,0.6));
#14849=CARTESIAN_POINT('',(3.8,-3.1,0.6));
#14850=CARTESIAN_POINT('',(14.,-1.9,0.6));
#14851=CARTESIAN_POINT('',(14.,-3.1,0.6));
#14852=CARTESIAN_POINT('',(3.8,-1.9,0.6));
#14853=CARTESIAN_POINT('',(14.,-1.9,0.6));
#14854=CARTESIAN_POINT('',(1.,1.,0.6));
#14855=CARTESIAN_POINT('',(3.8,-1.9,0.6));
#14856=CARTESIAN_POINT('',(1.,1.,0.6));
#14857=CARTESIAN_POINT('Origin',(0.,-1.,0.));
#14858=CARTESIAN_POINT('',(3.8,-3.1,0.));
#14859=CARTESIAN_POINT('',(0.,-1.,0.));
#14860=CARTESIAN_POINT('',(3.8,-3.1,0.));
#14861=CARTESIAN_POINT('Origin',(1.,1.,0.));
#14862=CARTESIAN_POINT('',(1.,1.,0.));
#14863=CARTESIAN_POINT('',(1.,1.,0.));
#14864=CARTESIAN_POINT('',(1.,1.,0.));
#14865=CARTESIAN_POINT('Origin',(3.8,-1.9,0.));
#14866=CARTESIAN_POINT('',(3.8,-1.9,0.));
#14867=CARTESIAN_POINT('',(3.8,-1.9,0.));
#14868=CARTESIAN_POINT('',(3.8,-1.9,0.));
#14869=CARTESIAN_POINT('Origin',(14.,-1.9,0.));
#14870=CARTESIAN_POINT('',(14.,-1.9,0.));
#14871=CARTESIAN_POINT('',(14.,-1.9,0.));
#14872=CARTESIAN_POINT('',(14.,-1.9,0.));
#14873=CARTESIAN_POINT('Origin',(14.,-3.1,0.));
#14874=CARTESIAN_POINT('',(14.,-3.1,0.));
#14875=CARTESIAN_POINT('',(14.,-3.1,0.));
#14876=CARTESIAN_POINT('',(14.,-3.1,0.));
#14877=CARTESIAN_POINT('Origin',(3.8,-3.1,0.));
#14878=CARTESIAN_POINT('',(3.8,-3.1,0.));
#14879=CARTESIAN_POINT('Origin',(0.,0.,0.));
#24786=UNCERTAINTY_MEASURE_WITH_UNIT(LENGTH_MEASURE(0.001),#24810,
'DISTANCE_ACCURACY_VALUE',
'Maximum model space distance between geometric entities at asserted c
onnectivities');
#24796=UNCERTAINTY_MEASURE_WITH_UNIT(LENGTH_MEASURE(0.001),#24810,
'DISTANCE_ACCURACY_VALUE',
'Maximum model space distance between geometric entities at asserted c
onnectivities');
#24799=(
GEOMETRIC_REPRESENTATION_CONTEXT(3)
GLOBAL_UNCERTAINTY_ASSIGNED_CONTEXT((#24786))
GLOBAL_UNIT_ASSIGNED_CONTEXT((#24810,#24812,#24813))
REPRESENTATION_CONTEXT('','3D')
);
#24809=(
GEOMETRIC_REPRESENTATION_CONTEXT(3)
GLOBAL_UNCERTAINTY_ASSIGNED_CONTEXT((#24796))
GLOBAL_UNIT_ASSIGNED_CONTEXT((#24810,#24812,#24813))
REPRESENTATION_CONTEXT('','3D')
);
#24810=(
LENGTH_UNIT()
NAMED_UNIT(*)
SI_UNIT(.CENTI.,.METRE.)
);
#24812=(
NAMED_UNIT(*)
PLANE_ANGLE_UNIT()
SI_UNIT($,.RADIAN.)
);
#24813=(
NAMED_UNIT(*)
SI_UNIT($,.STERADIAN.)
SOLID_ANGLE_UNIT()
);
#24816=SHAPE_DEFINITION_REPRESENTATION(#24828,#24856);
#24828=PRODUCT_DEFINITION_SHAPE('',$,#24869);
#24856=SHAPE_REPRESENTATION('',(#10121),#24799);
#24866=PRODUCT_DEFINITION_CONTEXT('part definition',#24904,'design');
#24869=PRODUCT_DEFINITION('Moving jaw and handle',
'Moving jaw and handle',#24881,#24866);
#24881=PRODUCT_DEFINITION_FORMATION('',$,#24908);
#24904=APPLICATION_CONTEXT(
'Core Data for Automotive Mechanical Design Process');
#24905=PRODUCT_CONTEXT('part definition',#24904,'mechanical');
#24908=PRODUCT('Moving jaw and handle','Moving jaw and handle',$,(#24905));
#24919=PRESENTATION_STYLE_ASSIGNMENT((#24927));
#24927=SURFACE_STYLE_USAGE(.BOTH.,#24935);
#24935=SURFACE_SIDE_STYLE('',(#24943));
#24943=SURFACE_STYLE_FILL_AREA(#24951);
#24951=FILL_AREA_STYLE('Tool steel gray',(#24959));
#24959=FILL_AREA_STYLE_COLOUR('Tool steel gray',#24967);
#24967=COLOUR_RGB('Tool steel gray',0.607843137254902,0.643137254901961,
0.698039215686274);
ENDSEC;
END-ISO-10303-21;
